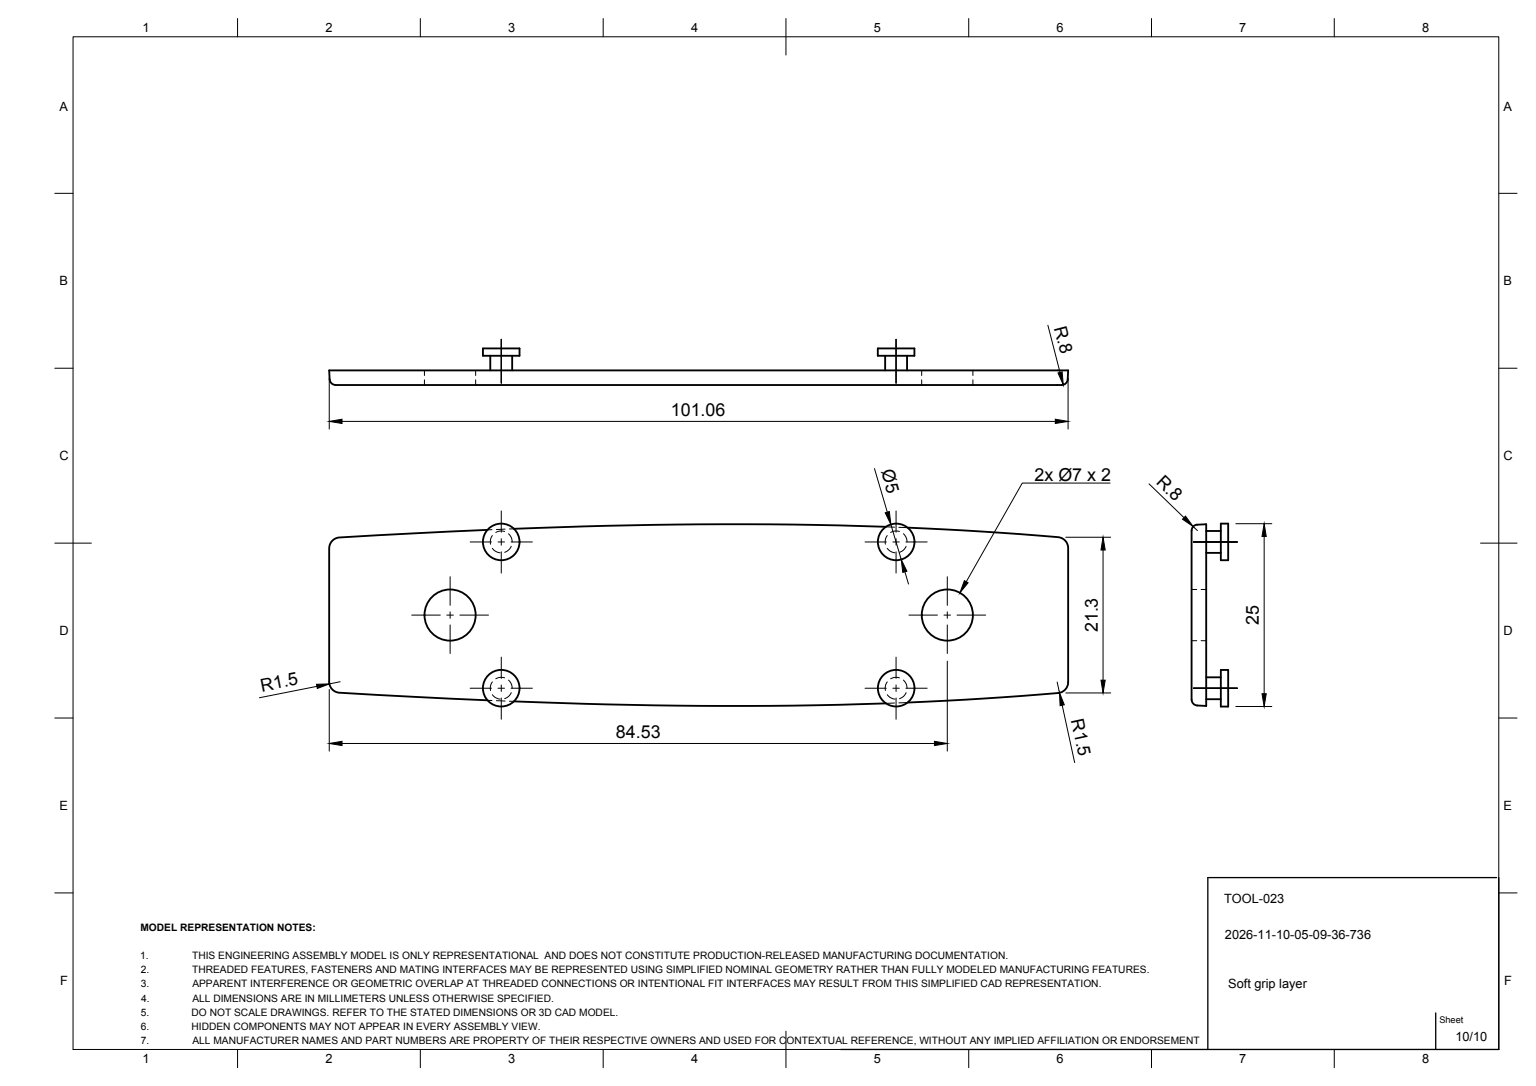
ISO-10303-21;
HEADER;
/* Generated by software containing ST-Developer
 * from STEP Tools, Inc. (www.steptools.com) 
 */

FILE_DESCRIPTION(
/* description */ (''),
/* implementation_level */ '2;1');

FILE_NAME(
/* name */ 'Soft grip layer.step',
/* time_stamp */ '2026-11-10T05:40:20-08:00',
/* author */ (''),
/* organization */ (''),
/* preprocessor_version */ 'ST-DEVELOPER v20.2',
/* originating_system */ 'Autodesk Translation Framework v15.17.0.0',
/* authorisation */ '');

FILE_SCHEMA (('AUTOMOTIVE_DESIGN { 1 0 10303 214 3 1 1 }'));
ENDSEC;

DATA;
#10=MECHANICAL_DESIGN_GEOMETRIC_PRESENTATION_REPRESENTATION('',(#579),#18580);
#160=B_SPLINE_SURFACE_WITH_KNOTS('',3,3,((#18008,#18009,#18010,#18011,#18012),
(#18013,#18014,#18015,#18016,#18017),(#18018,#18019,#18020,#18021,#18022),
(#18023,#18024,#18025,#18026,#18027),(#18028,#18029,#18030,#18031,#18032)),
 .UNSPECIFIED.,.F.,.F.,.F.,(4,1,4),(4,1,4),(0.,0.571428571428571,1.),(0.,
0.0453052401185593,0.105712226943305),.UNSPECIFIED.);
#161=B_SPLINE_SURFACE_WITH_KNOTS('',3,3,((#18055,#18056,#18057,#18058,#18059),
(#18060,#18061,#18062,#18063,#18064),(#18065,#18066,#18067,#18068,#18069),
(#18070,#18071,#18072,#18073,#18074),(#18075,#18076,#18077,#18078,#18079)),
 .UNSPECIFIED.,.F.,.F.,.F.,(4,1,4),(4,1,4),(0.,0.571428571428571,1.),(0.,
0.0453052401439183,0.105712227002476),.UNSPECIFIED.);
#162=B_SPLINE_SURFACE_WITH_KNOTS('',3,3,((#18093,#18094,#18095,#18096,#18097),
(#18098,#18099,#18100,#18101,#18102),(#18103,#18104,#18105,#18106,#18107),
(#18108,#18109,#18110,#18111,#18112),(#18113,#18114,#18115,#18116,#18117)),
 .UNSPECIFIED.,.F.,.F.,.F.,(4,1,4),(4,1,4),(0.,0.571428571428571,1.),(0.,
4.20509945658767,9.8118987320379),.UNSPECIFIED.);
#163=B_SPLINE_SURFACE_WITH_KNOTS('',3,3,((#18131,#18132,#18133,#18134,#18135),
(#18136,#18137,#18138,#18139,#18140),(#18141,#18142,#18143,#18144,#18145),
(#18146,#18147,#18148,#18149,#18150),(#18151,#18152,#18153,#18154,#18155)),
 .UNSPECIFIED.,.F.,.F.,.F.,(4,1,4),(4,1,4),(0.,0.571428571428571,1.),(0.,
0.0444882141544403,0.103805833027027),.UNSPECIFIED.);
#164=B_SPLINE_SURFACE_WITH_KNOTS('',3,3,((#18175,#18176,#18177,#18178,#18179),
(#18180,#18181,#18182,#18183,#18184),(#18185,#18186,#18187,#18188,#18189),
(#18190,#18191,#18192,#18193,#18194),(#18195,#18196,#18197,#18198,#18199)),
 .UNSPECIFIED.,.F.,.F.,.F.,(4,1,4),(4,1,4),(0.,0.571428571428571,1.),(2.06005858395869E-18,
0.0444882141931362,0.103805833117318),.UNSPECIFIED.);
#165=B_SPLINE_SURFACE_WITH_KNOTS('',3,3,((#18213,#18214,#18215,#18216,#18217),
(#18218,#18219,#18220,#18221,#18222),(#18223,#18224,#18225,#18226,#18227),
(#18228,#18229,#18230,#18231,#18232),(#18233,#18234,#18235,#18236,#18237)),
 .UNSPECIFIED.,.F.,.F.,.F.,(4,1,4),(4,1,4),(0.,0.571428571428571,1.),(0.,
4.20509909783593,9.81189789495051),.UNSPECIFIED.);
#166=B_SPLINE_SURFACE_WITH_KNOTS('',3,3,((#18260,#18261,#18262,#18263),
(#18264,#18265,#18266,#18267),(#18268,#18269,#18270,#18271),(#18272,#18273,
#18274,#18275),(#18276,#18277,#18278,#18279)),.UNSPECIFIED.,.F.,.F.,.F.,
(4,1,4),(4,4),(0.,0.571428571428571,1.),(-0.00268702576369722,0.125151053668407),
 .UNSPECIFIED.);
#167=B_SPLINE_SURFACE_WITH_KNOTS('',3,3,((#18313,#18314,#18315,#18316),
(#18317,#18318,#18319,#18320),(#18321,#18322,#18323,#18324),(#18325,#18326,
#18327,#18328)),.UNSPECIFIED.,.F.,.F.,.F.,(4,4),(4,4),(0.0135518988075539,
0.986045335056424),(0.,0.622596671418298),.UNSPECIFIED.);
#168=B_SPLINE_SURFACE_WITH_KNOTS('',3,3,((#18338,#18339,#18340,#18341),
(#18342,#18343,#18344,#18345),(#18346,#18347,#18348,#18349),(#18350,#18351,
#18352,#18353),(#18354,#18355,#18356,#18357)),.UNSPECIFIED.,.F.,.F.,.F.,
(4,1,4),(4,4),(0.,0.571428571428571,1.),(-0.00281084541253883,0.124959300034279),
 .UNSPECIFIED.);
#169=B_SPLINE_SURFACE_WITH_KNOTS('',3,3,((#18399,#18400,#18401,#18402),
(#18403,#18404,#18405,#18406),(#18407,#18408,#18409,#18410),(#18411,#18412,
#18413,#18414),(#18415,#18416,#18417,#18418)),.UNSPECIFIED.,.F.,.F.,.F.,
(4,1,4),(4,4),(0.,0.571428571428571,1.),(-0.00261432509268751,0.125151053668407),
 .UNSPECIFIED.);
#170=B_SPLINE_SURFACE_WITH_KNOTS('',3,3,((#18452,#18453,#18454,#18455),
(#18456,#18457,#18458,#18459),(#18460,#18461,#18462,#18463),(#18464,#18465,
#18466,#18467),(#18468,#18469,#18470,#18471)),.UNSPECIFIED.,.F.,.F.,.F.,
(4,1,4),(4,4),(0.,0.571428571428571,1.),(-0.00286362952972032,0.124959300034279),
 .UNSPECIFIED.);
#171=B_SPLINE_SURFACE_WITH_KNOTS('',3,3,((#18510,#18511,#18512,#18513),
(#18514,#18515,#18516,#18517),(#18518,#18519,#18520,#18521),(#18522,#18523,
#18524,#18525)),.UNSPECIFIED.,.F.,.F.,.F.,(4,4),(4,4),(0.0139546649435754,
0.986448101192446),(0.,0.622596671418299),.UNSPECIFIED.);
#528=B_SPLINE_CURVE_WITH_KNOTS('',3,(#18037,#18038,#18039,#18040,#18041),
 .UNSPECIFIED.,.F.,.F.,(4,1,4),(-0.105712226943305,-0.0453052401185593,
0.),.UNSPECIFIED.);
#529=B_SPLINE_CURVE_WITH_KNOTS('',3,(#18044,#18045,#18046,#18047,#18048),
 .UNSPECIFIED.,.F.,.F.,(4,1,4),(0.,0.0453052401185593,0.105712226943305),
 .UNSPECIFIED.);
#530=B_SPLINE_CURVE_WITH_KNOTS('',3,(#18083,#18084,#18085,#18086,#18087),
 .UNSPECIFIED.,.F.,.F.,(4,1,4),(-0.105712227002476,-0.0453052401439183,
0.),.UNSPECIFIED.);
#531=B_SPLINE_CURVE_WITH_KNOTS('',3,(#18088,#18089,#18090,#18091,#18092),
 .UNSPECIFIED.,.F.,.F.,(4,1,4),(0.,0.0453052401439183,0.105712227002476),
 .UNSPECIFIED.);
#532=B_SPLINE_CURVE_WITH_KNOTS('',3,(#18121,#18122,#18123,#18124,#18125),
 .UNSPECIFIED.,.F.,.F.,(4,1,4),(-9.8118987320379,-4.20509945658767,0.),
 .UNSPECIFIED.);
#533=B_SPLINE_CURVE_WITH_KNOTS('',3,(#18126,#18127,#18128,#18129,#18130),
 .UNSPECIFIED.,.F.,.F.,(4,1,4),(0.,4.20509945658767,9.8118987320379),
 .UNSPECIFIED.);
#534=B_SPLINE_CURVE_WITH_KNOTS('',3,(#18159,#18160,#18161,#18162,#18163),
 .UNSPECIFIED.,.F.,.F.,(4,1,4),(-0.103805833027027,-0.0444882141544403,
0.),.UNSPECIFIED.);
#535=B_SPLINE_CURVE_WITH_KNOTS('',3,(#18164,#18165,#18166,#18167,#18168),
 .UNSPECIFIED.,.F.,.F.,(4,1,4),(0.,0.0444882141544403,0.103805833027027),
 .UNSPECIFIED.);
#536=B_SPLINE_CURVE_WITH_KNOTS('',3,(#18203,#18204,#18205,#18206,#18207),
 .UNSPECIFIED.,.F.,.F.,(4,1,4),(-0.103805833117318,-0.0444882141931362,
-2.06005858395869E-18),.UNSPECIFIED.);
#537=B_SPLINE_CURVE_WITH_KNOTS('',3,(#18208,#18209,#18210,#18211,#18212),
 .UNSPECIFIED.,.F.,.F.,(4,1,4),(2.06005858395869E-18,0.0444882141931362,
0.103805833117318),.UNSPECIFIED.);
#538=B_SPLINE_CURVE_WITH_KNOTS('',3,(#18238,#18239,#18240,#18241,#18242),
 .UNSPECIFIED.,.F.,.F.,(4,1,4),(-9.81189789495051,-4.20509909783593,0.),
 .UNSPECIFIED.);
#539=B_SPLINE_CURVE_WITH_KNOTS('',3,(#18243,#18244,#18245,#18246,#18247),
 .UNSPECIFIED.,.F.,.F.,(4,1,4),(0.,4.20509909783593,9.81189789495051),
 .UNSPECIFIED.);
#540=B_SPLINE_CURVE_WITH_KNOTS('',3,(#18250,#18251,#18252,#18253),
 .UNSPECIFIED.,.F.,.F.,(4,4),(0.00062434729305816,0.125151053668407),
 .UNSPECIFIED.);
#541=B_SPLINE_CURVE_WITH_KNOTS('',3,(#18256,#18257,#18258,#18259),
 .UNSPECIFIED.,.F.,.F.,(4,4),(-0.125151053668407,-0.000624347293058304),
 .UNSPECIFIED.);
#542=B_SPLINE_CURVE_WITH_KNOTS('',3,(#18281,#18282,#18283,#18284),
 .UNSPECIFIED.,.F.,.F.,(4,4),(-0.124859357077656,3.91613824701764E-16),
 .UNSPECIFIED.);
#543=B_SPLINE_CURVE_WITH_KNOTS('',3,(#18285,#18286,#18287,#18288,#18289,
#18290,#18291,#18292,#18293,#18294,#18295,#18296,#18297,#18298,#18299,#18300,
#18301,#18302,#18303,#18304,#18305,#18306,#18307,#18308,#18309,#18310,#18311,
#18312),.UNSPECIFIED.,.F.,.F.,(4,3,3,3,3,3,3,3,3,4),(0.,0.0322709922822142,
0.0586131010579366,0.0908535483049993,0.095660418056781,0.117090121226367,
0.14947943031994,0.17008966569926,0.202270498561131,0.223122165115773),
 .UNSPECIFIED.);
#544=B_SPLINE_CURVE_WITH_KNOTS('',3,(#18330,#18331,#18332,#18333),
 .UNSPECIFIED.,.F.,.F.,(4,4),(1.57426155444895E-16,0.124757292074316),
 .UNSPECIFIED.);
#545=B_SPLINE_CURVE_WITH_KNOTS('',3,(#18334,#18335,#18336,#18337),
 .UNSPECIFIED.,.F.,.F.,(4,4),(0.0135518988075539,0.986045335056425),
 .UNSPECIFIED.);
#546=B_SPLINE_CURVE_WITH_KNOTS('',3,(#18359,#18360,#18361,#18362),
 .UNSPECIFIED.,.F.,.F.,(4,4),(-0.124959300034279,-0.000432357919845506),
 .UNSPECIFIED.);
#547=B_SPLINE_CURVE_WITH_KNOTS('',3,(#18363,#18364,#18365,#18366,#18367,
#18368,#18369,#18370,#18371,#18372,#18373,#18374,#18375,#18376,#18377,#18378,
#18379,#18380,#18381,#18382,#18383,#18384,#18385,#18386,#18387,#18388,#18389,
#18390),.UNSPECIFIED.,.F.,.F.,(4,3,3,3,3,3,3,3,3,4),(0.,0.0322720371751271,
0.0586511315716134,0.0908889384397039,0.0974306796249642,0.117149930269381,
0.149553095257184,0.172178760978465,0.204364325027201,0.227238249760569),
 .UNSPECIFIED.);
#548=B_SPLINE_CURVE_WITH_KNOTS('',3,(#18394,#18395,#18396,#18397),
 .UNSPECIFIED.,.F.,.F.,(4,4),(0.000432357919845864,0.124959300034279),
 .UNSPECIFIED.);
#549=B_SPLINE_CURVE_WITH_KNOTS('',3,(#18420,#18421,#18422,#18423,#18424,
#18425,#18426,#18427,#18428,#18429,#18430,#18431,#18432,#18433,#18434,#18435,
#18436,#18437,#18438,#18439,#18440,#18441,#18442,#18443,#18444,#18445,#18446,
#18447),.UNSPECIFIED.,.F.,.F.,(4,3,3,3,3,3,3,3,3,4),(0.,0.0322770007607458,
0.0586509099358757,0.0908890592373506,0.0956758252683957,0.117149647541228,
0.149540928065794,0.17012301918783,0.202296660223156,0.2231241621482),
 .UNSPECIFIED.);
#550=B_SPLINE_CURVE_WITH_KNOTS('',3,(#18448,#18449,#18450,#18451),
 .UNSPECIFIED.,.F.,.F.,(4,4),(1.94722710178397E-16,0.124859357077656),
 .UNSPECIFIED.);
#551=B_SPLINE_CURVE_WITH_KNOTS('',3,(#18473,#18474,#18475,#18476),
 .UNSPECIFIED.,.F.,.F.,(4,4),(-0.124757292074297,-2.43294967505747E-16),
 .UNSPECIFIED.);
#552=B_SPLINE_CURVE_WITH_KNOTS('',3,(#18477,#18478,#18479,#18480,#18481,
#18482,#18483,#18484,#18485,#18486,#18487,#18488,#18489,#18490,#18491,#18492,
#18493,#18494,#18495,#18496,#18497,#18498,#18499,#18500,#18501,#18502,#18503,
#18504),.UNSPECIFIED.,.F.,.F.,(4,3,3,3,3,3,3,3,3,4),(0.,0.0322677829554273,
0.0586251784806003,0.0908644978360146,0.097419835848357,0.117108565494702,
0.149510109206484,0.172155480916619,0.204345933772221,0.227236831322489),
 .UNSPECIFIED.);
#553=B_SPLINE_CURVE_WITH_KNOTS('',3,(#18506,#18507,#18508,#18509),
 .UNSPECIFIED.,.F.,.F.,(4,4),(0.0139546649435756,0.986448101192446),
 .UNSPECIFIED.);
#561=SHAPE_REPRESENTATION_RELATIONSHIP('SRR','None',#18632,#570);
#570=ADVANCED_BREP_SHAPE_REPRESENTATION('',(#588),#18578);
#579=STYLED_ITEM('',(#18688),#588);
#588=MANIFOLD_SOLID_BREP('Body1',#6551);
#637=FACE_BOUND('',#1558,.T.);
#638=FACE_BOUND('',#1562,.T.);
#639=FACE_BOUND('',#1566,.T.);
#640=FACE_BOUND('',#1570,.T.);
#641=FACE_BOUND('',#1590,.T.);
#642=FACE_BOUND('',#1591,.T.);
#643=FACE_BOUND('',#1596,.T.);
#644=FACE_BOUND('',#1597,.T.);
#645=FACE_BOUND('',#1598,.T.);
#646=FACE_BOUND('',#1599,.T.);
#647=FACE_BOUND('',#1600,.T.);
#648=FACE_BOUND('',#1601,.T.);
#782=PLANE('',#7063);
#783=PLANE('',#7068);
#784=PLANE('',#7069);
#785=PLANE('',#7074);
#786=PLANE('',#7075);
#787=PLANE('',#7080);
#788=PLANE('',#7081);
#789=PLANE('',#7086);
#790=PLANE('',#7105);
#791=PLANE('',#7106);
#792=PLANE('',#7107);
#793=PLANE('',#7108);
#1132=FACE_OUTER_BOUND('',#1555,.T.);
#1133=FACE_OUTER_BOUND('',#1556,.T.);
#1134=FACE_OUTER_BOUND('',#1557,.T.);
#1135=FACE_OUTER_BOUND('',#1559,.T.);
#1136=FACE_OUTER_BOUND('',#1560,.T.);
#1137=FACE_OUTER_BOUND('',#1561,.T.);
#1138=FACE_OUTER_BOUND('',#1563,.T.);
#1139=FACE_OUTER_BOUND('',#1564,.T.);
#1140=FACE_OUTER_BOUND('',#1565,.T.);
#1141=FACE_OUTER_BOUND('',#1567,.T.);
#1142=FACE_OUTER_BOUND('',#1568,.T.);
#1143=FACE_OUTER_BOUND('',#1569,.T.);
#1144=FACE_OUTER_BOUND('',#1571,.T.);
#1145=FACE_OUTER_BOUND('',#1572,.T.);
#1146=FACE_OUTER_BOUND('',#1573,.T.);
#1147=FACE_OUTER_BOUND('',#1574,.T.);
#1148=FACE_OUTER_BOUND('',#1575,.T.);
#1149=FACE_OUTER_BOUND('',#1576,.T.);
#1150=FACE_OUTER_BOUND('',#1577,.T.);
#1151=FACE_OUTER_BOUND('',#1578,.T.);
#1152=FACE_OUTER_BOUND('',#1579,.T.);
#1153=FACE_OUTER_BOUND('',#1580,.T.);
#1154=FACE_OUTER_BOUND('',#1581,.T.);
#1155=FACE_OUTER_BOUND('',#1582,.T.);
#1156=FACE_OUTER_BOUND('',#1583,.T.);
#1157=FACE_OUTER_BOUND('',#1584,.T.);
#1158=FACE_OUTER_BOUND('',#1585,.T.);
#1159=FACE_OUTER_BOUND('',#1586,.T.);
#1160=FACE_OUTER_BOUND('',#1587,.T.);
#1161=FACE_OUTER_BOUND('',#1588,.T.);
#1162=FACE_OUTER_BOUND('',#1589,.T.);
#1163=FACE_OUTER_BOUND('',#1592,.T.);
#1164=FACE_OUTER_BOUND('',#1593,.T.);
#1165=FACE_OUTER_BOUND('',#1594,.T.);
#1166=FACE_OUTER_BOUND('',#1595,.T.);
#1167=FACE_OUTER_BOUND('',#1602,.T.);
#1555=EDGE_LOOP('',(#5882,#5883,#5884,#5885));
#1556=EDGE_LOOP('',(#5886,#5887,#5888,#5889));
#1557=EDGE_LOOP('',(#5890));
#1558=EDGE_LOOP('',(#5891));
#1559=EDGE_LOOP('',(#5892,#5893,#5894,#5895));
#1560=EDGE_LOOP('',(#5896));
#1561=EDGE_LOOP('',(#5897));
#1562=EDGE_LOOP('',(#5898));
#1563=EDGE_LOOP('',(#5899,#5900,#5901,#5902));
#1564=EDGE_LOOP('',(#5903));
#1565=EDGE_LOOP('',(#5904));
#1566=EDGE_LOOP('',(#5905));
#1567=EDGE_LOOP('',(#5906,#5907,#5908,#5909));
#1568=EDGE_LOOP('',(#5910));
#1569=EDGE_LOOP('',(#5911));
#1570=EDGE_LOOP('',(#5912));
#1571=EDGE_LOOP('',(#5913,#5914,#5915,#5916));
#1572=EDGE_LOOP('',(#5917));
#1573=EDGE_LOOP('',(#5918,#5919,#5920,#5921));
#1574=EDGE_LOOP('',(#5922,#5923,#5924,#5925));
#1575=EDGE_LOOP('',(#5926,#5927,#5928,#5929));
#1576=EDGE_LOOP('',(#5930,#5931,#5932,#5933));
#1577=EDGE_LOOP('',(#5934,#5935,#5936,#5937));
#1578=EDGE_LOOP('',(#5938,#5939,#5940,#5941));
#1579=EDGE_LOOP('',(#5942,#5943,#5944,#5945));
#1580=EDGE_LOOP('',(#5946,#5947,#5948,#5949));
#1581=EDGE_LOOP('',(#5950,#5951,#5952,#5953));
#1582=EDGE_LOOP('',(#5954,#5955,#5956,#5957));
#1583=EDGE_LOOP('',(#5958,#5959,#5960,#5961));
#1584=EDGE_LOOP('',(#5962,#5963,#5964,#5965));
#1585=EDGE_LOOP('',(#5966,#5967,#5968,#5969));
#1586=EDGE_LOOP('',(#5970,#5971,#5972,#5973));
#1587=EDGE_LOOP('',(#5974,#5975,#5976,#5977));
#1588=EDGE_LOOP('',(#5978,#5979,#5980,#5981));
#1589=EDGE_LOOP('',(#5982,#5983,#5984,#5985,#5986,#5987,#5988,#5989));
#1590=EDGE_LOOP('',(#5990));
#1591=EDGE_LOOP('',(#5991));
#1592=EDGE_LOOP('',(#5992,#5993,#5994,#5995));
#1593=EDGE_LOOP('',(#5996,#5997,#5998,#5999));
#1594=EDGE_LOOP('',(#6000,#6001,#6002,#6003));
#1595=EDGE_LOOP('',(#6004,#6005,#6006,#6007,#6008,#6009,#6010,#6011));
#1596=EDGE_LOOP('',(#6012));
#1597=EDGE_LOOP('',(#6013));
#1598=EDGE_LOOP('',(#6014));
#1599=EDGE_LOOP('',(#6015));
#1600=EDGE_LOOP('',(#6016));
#1601=EDGE_LOOP('',(#6017));
#1602=EDGE_LOOP('',(#6018,#6019,#6020,#6021));
#1998=LINE('',#17944,#2405);
#1999=LINE('',#17950,#2406);
#2000=LINE('',#17960,#2407);
#2001=LINE('',#17970,#2408);
#2002=LINE('',#17980,#2409);
#2003=LINE('',#17990,#2410);
#2004=LINE('',#17994,#2411);
#2005=LINE('',#17998,#2412);
#2006=LINE('',#18002,#2413);
#2007=LINE('',#18006,#2414);
#2008=LINE('',#18053,#2415);
#2009=LINE('',#18054,#2416);
#2010=LINE('',#18173,#2417);
#2011=LINE('',#18174,#2418);
#2012=LINE('',#18255,#2419);
#2013=LINE('',#18398,#2420);
#2405=VECTOR('',#8335,0.35);
#2406=VECTOR('',#8342,0.35);
#2407=VECTOR('',#8355,0.25);
#2408=VECTOR('',#8368,0.25);
#2409=VECTOR('',#8381,0.25);
#2410=VECTOR('',#8394,0.25);
#2411=VECTOR('',#8399,0.15);
#2412=VECTOR('',#8404,0.15);
#2413=VECTOR('',#8409,0.15);
#2414=VECTOR('',#8414,0.15);
#2415=VECTOR('',#8425,1.);
#2416=VECTOR('',#8426,1.);
#2417=VECTOR('',#8437,1.);
#2418=VECTOR('',#8438,1.);
#2419=VECTOR('',#8443,1.);
#2420=VECTOR('',#8448,1.);
#2549=CIRCLE('',#7058,0.35);
#2550=CIRCLE('',#7059,0.35);
#2551=CIRCLE('',#7061,0.35);
#2552=CIRCLE('',#7062,0.35);
#2553=CIRCLE('',#7064,0.25);
#2554=CIRCLE('',#7065,0.15);
#2555=CIRCLE('',#7067,0.25);
#2556=CIRCLE('',#7070,0.25);
#2557=CIRCLE('',#7071,0.15);
#2558=CIRCLE('',#7073,0.25);
#2559=CIRCLE('',#7076,0.25);
#2560=CIRCLE('',#7077,0.15);
#2561=CIRCLE('',#7079,0.25);
#2562=CIRCLE('',#7082,0.25);
#2563=CIRCLE('',#7083,0.15);
#2564=CIRCLE('',#7085,0.25);
#2565=CIRCLE('',#7088,0.15);
#2566=CIRCLE('',#7090,0.15);
#2567=CIRCLE('',#7092,0.15);
#2568=CIRCLE('',#7094,0.15);
#2569=CIRCLE('',#7095,0.0800000000000001);
#2570=CIRCLE('',#7096,0.0799999999999999);
#2571=CIRCLE('',#7098,0.0800000000000001);
#2572=CIRCLE('',#7099,0.0800000000000001);
#2573=CIRCLE('',#7100,0.0800000000000001);
#2574=CIRCLE('',#7101,0.0800000000000001);
#2575=CIRCLE('',#7103,0.0800000000000001);
#2576=CIRCLE('',#7104,0.0800000000000001);
#3145=VERTEX_POINT('',#17941);
#3146=VERTEX_POINT('',#17943);
#3147=VERTEX_POINT('',#17947);
#3148=VERTEX_POINT('',#17949);
#3149=VERTEX_POINT('',#17953);
#3150=VERTEX_POINT('',#17955);
#3151=VERTEX_POINT('',#17958);
#3152=VERTEX_POINT('',#17963);
#3153=VERTEX_POINT('',#17965);
#3154=VERTEX_POINT('',#17968);
#3155=VERTEX_POINT('',#17973);
#3156=VERTEX_POINT('',#17975);
#3157=VERTEX_POINT('',#17978);
#3158=VERTEX_POINT('',#17983);
#3159=VERTEX_POINT('',#17985);
#3160=VERTEX_POINT('',#17988);
#3161=VERTEX_POINT('',#17993);
#3162=VERTEX_POINT('',#17997);
#3163=VERTEX_POINT('',#18001);
#3164=VERTEX_POINT('',#18005);
#3165=VERTEX_POINT('',#18033);
#3166=VERTEX_POINT('',#18034);
#3167=VERTEX_POINT('',#18036);
#3168=VERTEX_POINT('',#18042);
#3169=VERTEX_POINT('',#18050);
#3170=VERTEX_POINT('',#18051);
#3171=VERTEX_POINT('',#18080);
#3172=VERTEX_POINT('',#18081);
#3173=VERTEX_POINT('',#18118);
#3174=VERTEX_POINT('',#18119);
#3175=VERTEX_POINT('',#18156);
#3176=VERTEX_POINT('',#18157);
#3177=VERTEX_POINT('',#18170);
#3178=VERTEX_POINT('',#18171);
#3179=VERTEX_POINT('',#18200);
#3180=VERTEX_POINT('',#18201);
#3181=VERTEX_POINT('',#18249);
#3182=VERTEX_POINT('',#18254);
#3183=VERTEX_POINT('',#18280);
#3184=VERTEX_POINT('',#18329);
#3185=VERTEX_POINT('',#18358);
#3186=VERTEX_POINT('',#18393);
#3187=VERTEX_POINT('',#18419);
#3188=VERTEX_POINT('',#18472);
#4064=EDGE_CURVE('',#3145,#3145,#2549,.T.);
#4065=EDGE_CURVE('',#3145,#3146,#1998,.T.);
#4066=EDGE_CURVE('',#3146,#3146,#2550,.T.);
#4067=EDGE_CURVE('',#3147,#3147,#2551,.T.);
#4068=EDGE_CURVE('',#3147,#3148,#1999,.T.);
#4069=EDGE_CURVE('',#3148,#3148,#2552,.T.);
#4070=EDGE_CURVE('',#3149,#3149,#2553,.T.);
#4071=EDGE_CURVE('',#3150,#3150,#2554,.T.);
#4072=EDGE_CURVE('',#3151,#3151,#2555,.T.);
#4073=EDGE_CURVE('',#3151,#3149,#2000,.T.);
#4074=EDGE_CURVE('',#3152,#3152,#2556,.T.);
#4075=EDGE_CURVE('',#3153,#3153,#2557,.T.);
#4076=EDGE_CURVE('',#3154,#3154,#2558,.T.);
#4077=EDGE_CURVE('',#3154,#3152,#2001,.T.);
#4078=EDGE_CURVE('',#3155,#3155,#2559,.T.);
#4079=EDGE_CURVE('',#3156,#3156,#2560,.T.);
#4080=EDGE_CURVE('',#3157,#3157,#2561,.T.);
#4081=EDGE_CURVE('',#3157,#3155,#2002,.T.);
#4082=EDGE_CURVE('',#3158,#3158,#2562,.T.);
#4083=EDGE_CURVE('',#3159,#3159,#2563,.T.);
#4084=EDGE_CURVE('',#3160,#3160,#2564,.T.);
#4085=EDGE_CURVE('',#3160,#3158,#2003,.T.);
#4086=EDGE_CURVE('',#3150,#3161,#2004,.T.);
#4087=EDGE_CURVE('',#3161,#3161,#2565,.T.);
#4088=EDGE_CURVE('',#3153,#3162,#2005,.T.);
#4089=EDGE_CURVE('',#3162,#3162,#2566,.T.);
#4090=EDGE_CURVE('',#3156,#3163,#2006,.T.);
#4091=EDGE_CURVE('',#3163,#3163,#2567,.T.);
#4092=EDGE_CURVE('',#3159,#3164,#2007,.T.);
#4093=EDGE_CURVE('',#3164,#3164,#2568,.T.);
#4094=EDGE_CURVE('',#3165,#3166,#2569,.T.);
#4095=EDGE_CURVE('',#3166,#3167,#528,.T.);
#4096=EDGE_CURVE('',#3167,#3168,#2570,.T.);
#4097=EDGE_CURVE('',#3168,#3165,#529,.T.);
#4098=EDGE_CURVE('',#3169,#3170,#2571,.T.);
#4099=EDGE_CURVE('',#3170,#3166,#2008,.T.);
#4100=EDGE_CURVE('',#3165,#3169,#2009,.T.);
#4101=EDGE_CURVE('',#3171,#3172,#2572,.T.);
#4102=EDGE_CURVE('',#3172,#3170,#530,.T.);
#4103=EDGE_CURVE('',#3169,#3171,#531,.T.);
#4104=EDGE_CURVE('',#3173,#3174,#2573,.T.);
#4105=EDGE_CURVE('',#3174,#3172,#532,.T.);
#4106=EDGE_CURVE('',#3171,#3173,#533,.T.);
#4107=EDGE_CURVE('',#3175,#3176,#2574,.T.);
#4108=EDGE_CURVE('',#3176,#3174,#534,.T.);
#4109=EDGE_CURVE('',#3173,#3175,#535,.T.);
#4110=EDGE_CURVE('',#3177,#3178,#2575,.T.);
#4111=EDGE_CURVE('',#3178,#3176,#2010,.T.);
#4112=EDGE_CURVE('',#3175,#3177,#2011,.T.);
#4113=EDGE_CURVE('',#3179,#3180,#2576,.T.);
#4114=EDGE_CURVE('',#3180,#3178,#536,.T.);
#4115=EDGE_CURVE('',#3177,#3179,#537,.T.);
#4116=EDGE_CURVE('',#3167,#3180,#538,.T.);
#4117=EDGE_CURVE('',#3179,#3168,#539,.T.);
#4118=EDGE_CURVE('',#3181,#3178,#540,.T.);
#4119=EDGE_CURVE('',#3182,#3181,#2012,.T.);
#4120=EDGE_CURVE('',#3176,#3182,#541,.T.);
#4121=EDGE_CURVE('',#3180,#3183,#542,.T.);
#4122=EDGE_CURVE('',#3183,#3181,#543,.T.);
#4123=EDGE_CURVE('',#3184,#3167,#544,.T.);
#4124=EDGE_CURVE('',#3183,#3184,#545,.T.);
#4125=EDGE_CURVE('',#3166,#3185,#546,.T.);
#4126=EDGE_CURVE('',#3185,#3184,#547,.T.);
#4127=EDGE_CURVE('',#3186,#3170,#548,.T.);
#4128=EDGE_CURVE('',#3185,#3186,#2013,.T.);
#4129=EDGE_CURVE('',#3182,#3187,#549,.T.);
#4130=EDGE_CURVE('',#3187,#3174,#550,.T.);
#4131=EDGE_CURVE('',#3172,#3188,#551,.T.);
#4132=EDGE_CURVE('',#3188,#3186,#552,.T.);
#4133=EDGE_CURVE('',#3188,#3187,#553,.T.);
#5882=ORIENTED_EDGE('',*,*,#4064,.F.);
#5883=ORIENTED_EDGE('',*,*,#4065,.T.);
#5884=ORIENTED_EDGE('',*,*,#4066,.F.);
#5885=ORIENTED_EDGE('',*,*,#4065,.F.);
#5886=ORIENTED_EDGE('',*,*,#4067,.F.);
#5887=ORIENTED_EDGE('',*,*,#4068,.T.);
#5888=ORIENTED_EDGE('',*,*,#4069,.F.);
#5889=ORIENTED_EDGE('',*,*,#4068,.F.);
#5890=ORIENTED_EDGE('',*,*,#4070,.T.);
#5891=ORIENTED_EDGE('',*,*,#4071,.T.);
#5892=ORIENTED_EDGE('',*,*,#4072,.F.);
#5893=ORIENTED_EDGE('',*,*,#4073,.T.);
#5894=ORIENTED_EDGE('',*,*,#4070,.F.);
#5895=ORIENTED_EDGE('',*,*,#4073,.F.);
#5896=ORIENTED_EDGE('',*,*,#4072,.T.);
#5897=ORIENTED_EDGE('',*,*,#4074,.T.);
#5898=ORIENTED_EDGE('',*,*,#4075,.T.);
#5899=ORIENTED_EDGE('',*,*,#4076,.F.);
#5900=ORIENTED_EDGE('',*,*,#4077,.T.);
#5901=ORIENTED_EDGE('',*,*,#4074,.F.);
#5902=ORIENTED_EDGE('',*,*,#4077,.F.);
#5903=ORIENTED_EDGE('',*,*,#4076,.T.);
#5904=ORIENTED_EDGE('',*,*,#4078,.T.);
#5905=ORIENTED_EDGE('',*,*,#4079,.T.);
#5906=ORIENTED_EDGE('',*,*,#4080,.F.);
#5907=ORIENTED_EDGE('',*,*,#4081,.T.);
#5908=ORIENTED_EDGE('',*,*,#4078,.F.);
#5909=ORIENTED_EDGE('',*,*,#4081,.F.);
#5910=ORIENTED_EDGE('',*,*,#4080,.T.);
#5911=ORIENTED_EDGE('',*,*,#4082,.T.);
#5912=ORIENTED_EDGE('',*,*,#4083,.T.);
#5913=ORIENTED_EDGE('',*,*,#4084,.F.);
#5914=ORIENTED_EDGE('',*,*,#4085,.T.);
#5915=ORIENTED_EDGE('',*,*,#4082,.F.);
#5916=ORIENTED_EDGE('',*,*,#4085,.F.);
#5917=ORIENTED_EDGE('',*,*,#4084,.T.);
#5918=ORIENTED_EDGE('',*,*,#4071,.F.);
#5919=ORIENTED_EDGE('',*,*,#4086,.T.);
#5920=ORIENTED_EDGE('',*,*,#4087,.F.);
#5921=ORIENTED_EDGE('',*,*,#4086,.F.);
#5922=ORIENTED_EDGE('',*,*,#4075,.F.);
#5923=ORIENTED_EDGE('',*,*,#4088,.T.);
#5924=ORIENTED_EDGE('',*,*,#4089,.F.);
#5925=ORIENTED_EDGE('',*,*,#4088,.F.);
#5926=ORIENTED_EDGE('',*,*,#4079,.F.);
#5927=ORIENTED_EDGE('',*,*,#4090,.T.);
#5928=ORIENTED_EDGE('',*,*,#4091,.F.);
#5929=ORIENTED_EDGE('',*,*,#4090,.F.);
#5930=ORIENTED_EDGE('',*,*,#4083,.F.);
#5931=ORIENTED_EDGE('',*,*,#4092,.T.);
#5932=ORIENTED_EDGE('',*,*,#4093,.F.);
#5933=ORIENTED_EDGE('',*,*,#4092,.F.);
#5934=ORIENTED_EDGE('',*,*,#4094,.T.);
#5935=ORIENTED_EDGE('',*,*,#4095,.T.);
#5936=ORIENTED_EDGE('',*,*,#4096,.T.);
#5937=ORIENTED_EDGE('',*,*,#4097,.T.);
#5938=ORIENTED_EDGE('',*,*,#4098,.T.);
#5939=ORIENTED_EDGE('',*,*,#4099,.T.);
#5940=ORIENTED_EDGE('',*,*,#4094,.F.);
#5941=ORIENTED_EDGE('',*,*,#4100,.T.);
#5942=ORIENTED_EDGE('',*,*,#4101,.T.);
#5943=ORIENTED_EDGE('',*,*,#4102,.T.);
#5944=ORIENTED_EDGE('',*,*,#4098,.F.);
#5945=ORIENTED_EDGE('',*,*,#4103,.T.);
#5946=ORIENTED_EDGE('',*,*,#4104,.T.);
#5947=ORIENTED_EDGE('',*,*,#4105,.T.);
#5948=ORIENTED_EDGE('',*,*,#4101,.F.);
#5949=ORIENTED_EDGE('',*,*,#4106,.T.);
#5950=ORIENTED_EDGE('',*,*,#4107,.T.);
#5951=ORIENTED_EDGE('',*,*,#4108,.T.);
#5952=ORIENTED_EDGE('',*,*,#4104,.F.);
#5953=ORIENTED_EDGE('',*,*,#4109,.T.);
#5954=ORIENTED_EDGE('',*,*,#4110,.T.);
#5955=ORIENTED_EDGE('',*,*,#4111,.T.);
#5956=ORIENTED_EDGE('',*,*,#4107,.F.);
#5957=ORIENTED_EDGE('',*,*,#4112,.T.);
#5958=ORIENTED_EDGE('',*,*,#4113,.T.);
#5959=ORIENTED_EDGE('',*,*,#4114,.T.);
#5960=ORIENTED_EDGE('',*,*,#4110,.F.);
#5961=ORIENTED_EDGE('',*,*,#4115,.T.);
#5962=ORIENTED_EDGE('',*,*,#4096,.F.);
#5963=ORIENTED_EDGE('',*,*,#4116,.T.);
#5964=ORIENTED_EDGE('',*,*,#4113,.F.);
#5965=ORIENTED_EDGE('',*,*,#4117,.T.);
#5966=ORIENTED_EDGE('',*,*,#4111,.F.);
#5967=ORIENTED_EDGE('',*,*,#4118,.F.);
#5968=ORIENTED_EDGE('',*,*,#4119,.F.);
#5969=ORIENTED_EDGE('',*,*,#4120,.F.);
#5970=ORIENTED_EDGE('',*,*,#4114,.F.);
#5971=ORIENTED_EDGE('',*,*,#4121,.T.);
#5972=ORIENTED_EDGE('',*,*,#4122,.T.);
#5973=ORIENTED_EDGE('',*,*,#4118,.T.);
#5974=ORIENTED_EDGE('',*,*,#4116,.F.);
#5975=ORIENTED_EDGE('',*,*,#4123,.F.);
#5976=ORIENTED_EDGE('',*,*,#4124,.F.);
#5977=ORIENTED_EDGE('',*,*,#4121,.F.);
#5978=ORIENTED_EDGE('',*,*,#4095,.F.);
#5979=ORIENTED_EDGE('',*,*,#4125,.T.);
#5980=ORIENTED_EDGE('',*,*,#4126,.T.);
#5981=ORIENTED_EDGE('',*,*,#4123,.T.);
#5982=ORIENTED_EDGE('',*,*,#4097,.F.);
#5983=ORIENTED_EDGE('',*,*,#4117,.F.);
#5984=ORIENTED_EDGE('',*,*,#4115,.F.);
#5985=ORIENTED_EDGE('',*,*,#4112,.F.);
#5986=ORIENTED_EDGE('',*,*,#4109,.F.);
#5987=ORIENTED_EDGE('',*,*,#4106,.F.);
#5988=ORIENTED_EDGE('',*,*,#4103,.F.);
#5989=ORIENTED_EDGE('',*,*,#4100,.F.);
#5990=ORIENTED_EDGE('',*,*,#4064,.T.);
#5991=ORIENTED_EDGE('',*,*,#4067,.T.);
#5992=ORIENTED_EDGE('',*,*,#4099,.F.);
#5993=ORIENTED_EDGE('',*,*,#4127,.F.);
#5994=ORIENTED_EDGE('',*,*,#4128,.F.);
#5995=ORIENTED_EDGE('',*,*,#4125,.F.);
#5996=ORIENTED_EDGE('',*,*,#4108,.F.);
#5997=ORIENTED_EDGE('',*,*,#4120,.T.);
#5998=ORIENTED_EDGE('',*,*,#4129,.T.);
#5999=ORIENTED_EDGE('',*,*,#4130,.T.);
#6000=ORIENTED_EDGE('',*,*,#4102,.F.);
#6001=ORIENTED_EDGE('',*,*,#4131,.T.);
#6002=ORIENTED_EDGE('',*,*,#4132,.T.);
#6003=ORIENTED_EDGE('',*,*,#4127,.T.);
#6004=ORIENTED_EDGE('',*,*,#4126,.F.);
#6005=ORIENTED_EDGE('',*,*,#4128,.T.);
#6006=ORIENTED_EDGE('',*,*,#4132,.F.);
#6007=ORIENTED_EDGE('',*,*,#4133,.T.);
#6008=ORIENTED_EDGE('',*,*,#4129,.F.);
#6009=ORIENTED_EDGE('',*,*,#4119,.T.);
#6010=ORIENTED_EDGE('',*,*,#4122,.F.);
#6011=ORIENTED_EDGE('',*,*,#4124,.T.);
#6012=ORIENTED_EDGE('',*,*,#4066,.T.);
#6013=ORIENTED_EDGE('',*,*,#4069,.T.);
#6014=ORIENTED_EDGE('',*,*,#4087,.T.);
#6015=ORIENTED_EDGE('',*,*,#4089,.T.);
#6016=ORIENTED_EDGE('',*,*,#4091,.T.);
#6017=ORIENTED_EDGE('',*,*,#4093,.T.);
#6018=ORIENTED_EDGE('',*,*,#4105,.F.);
#6019=ORIENTED_EDGE('',*,*,#4130,.F.);
#6020=ORIENTED_EDGE('',*,*,#4133,.F.);
#6021=ORIENTED_EDGE('',*,*,#4131,.F.);
#6154=CYLINDRICAL_SURFACE('',#7057,0.35);
#6155=CYLINDRICAL_SURFACE('',#7060,0.35);
#6156=CYLINDRICAL_SURFACE('',#7066,0.25);
#6157=CYLINDRICAL_SURFACE('',#7072,0.25);
#6158=CYLINDRICAL_SURFACE('',#7078,0.25);
#6159=CYLINDRICAL_SURFACE('',#7084,0.25);
#6160=CYLINDRICAL_SURFACE('',#7087,0.15);
#6161=CYLINDRICAL_SURFACE('',#7089,0.15);
#6162=CYLINDRICAL_SURFACE('',#7091,0.15);
#6163=CYLINDRICAL_SURFACE('',#7093,0.15);
#6164=CYLINDRICAL_SURFACE('',#7097,0.08);
#6165=CYLINDRICAL_SURFACE('',#7102,0.08);
#6504=ADVANCED_FACE('',(#1132),#6154,.F.);
#6505=ADVANCED_FACE('',(#1133),#6155,.F.);
#6506=ADVANCED_FACE('',(#1134,#637),#782,.T.);
#6507=ADVANCED_FACE('',(#1135),#6156,.T.);
#6508=ADVANCED_FACE('',(#1136),#783,.F.);
#6509=ADVANCED_FACE('',(#1137,#638),#784,.T.);
#6510=ADVANCED_FACE('',(#1138),#6157,.T.);
#6511=ADVANCED_FACE('',(#1139),#785,.F.);
#6512=ADVANCED_FACE('',(#1140,#639),#786,.T.);
#6513=ADVANCED_FACE('',(#1141),#6158,.T.);
#6514=ADVANCED_FACE('',(#1142),#787,.F.);
#6515=ADVANCED_FACE('',(#1143,#640),#788,.T.);
#6516=ADVANCED_FACE('',(#1144),#6159,.T.);
#6517=ADVANCED_FACE('',(#1145),#789,.F.);
#6518=ADVANCED_FACE('',(#1146),#6160,.T.);
#6519=ADVANCED_FACE('',(#1147),#6161,.T.);
#6520=ADVANCED_FACE('',(#1148),#6162,.T.);
#6521=ADVANCED_FACE('',(#1149),#6163,.T.);
#6522=ADVANCED_FACE('',(#1150),#160,.F.);
#6523=ADVANCED_FACE('',(#1151),#6164,.T.);
#6524=ADVANCED_FACE('',(#1152),#161,.F.);
#6525=ADVANCED_FACE('',(#1153),#162,.F.);
#6526=ADVANCED_FACE('',(#1154),#163,.F.);
#6527=ADVANCED_FACE('',(#1155),#6165,.T.);
#6528=ADVANCED_FACE('',(#1156),#164,.F.);
#6529=ADVANCED_FACE('',(#1157),#165,.F.);
#6530=ADVANCED_FACE('',(#1158),#790,.F.);
#6531=ADVANCED_FACE('',(#1159),#166,.F.);
#6532=ADVANCED_FACE('',(#1160),#167,.F.);
#6533=ADVANCED_FACE('',(#1161),#168,.F.);
#6534=ADVANCED_FACE('',(#1162,#641,#642),#791,.T.);
#6535=ADVANCED_FACE('',(#1163),#792,.F.);
#6536=ADVANCED_FACE('',(#1164),#169,.F.);
#6537=ADVANCED_FACE('',(#1165),#170,.F.);
#6538=ADVANCED_FACE('',(#1166,#643,#644,#645,#646,#647,#648),#793,.F.);
#6539=ADVANCED_FACE('',(#1167),#171,.F.);
#6551=CLOSED_SHELL('',(#6504,#6505,#6506,#6507,#6508,#6509,#6510,#6511,
#6512,#6513,#6514,#6515,#6516,#6517,#6518,#6519,#6520,#6521,#6522,#6523,
#6524,#6525,#6526,#6527,#6528,#6529,#6530,#6531,#6532,#6533,#6534,#6535,
#6536,#6537,#6538,#6539));
#7056=AXIS2_PLACEMENT_3D('',#17939,#8329,#8330);
#7057=AXIS2_PLACEMENT_3D('',#17940,#8331,#8332);
#7058=AXIS2_PLACEMENT_3D('',#17942,#8333,#8334);
#7059=AXIS2_PLACEMENT_3D('',#17945,#8336,#8337);
#7060=AXIS2_PLACEMENT_3D('',#17946,#8338,#8339);
#7061=AXIS2_PLACEMENT_3D('',#17948,#8340,#8341);
#7062=AXIS2_PLACEMENT_3D('',#17951,#8343,#8344);
#7063=AXIS2_PLACEMENT_3D('',#17952,#8345,#8346);
#7064=AXIS2_PLACEMENT_3D('',#17954,#8347,#8348);
#7065=AXIS2_PLACEMENT_3D('',#17956,#8349,#8350);
#7066=AXIS2_PLACEMENT_3D('',#17957,#8351,#8352);
#7067=AXIS2_PLACEMENT_3D('',#17959,#8353,#8354);
#7068=AXIS2_PLACEMENT_3D('',#17961,#8356,#8357);
#7069=AXIS2_PLACEMENT_3D('',#17962,#8358,#8359);
#7070=AXIS2_PLACEMENT_3D('',#17964,#8360,#8361);
#7071=AXIS2_PLACEMENT_3D('',#17966,#8362,#8363);
#7072=AXIS2_PLACEMENT_3D('',#17967,#8364,#8365);
#7073=AXIS2_PLACEMENT_3D('',#17969,#8366,#8367);
#7074=AXIS2_PLACEMENT_3D('',#17971,#8369,#8370);
#7075=AXIS2_PLACEMENT_3D('',#17972,#8371,#8372);
#7076=AXIS2_PLACEMENT_3D('',#17974,#8373,#8374);
#7077=AXIS2_PLACEMENT_3D('',#17976,#8375,#8376);
#7078=AXIS2_PLACEMENT_3D('',#17977,#8377,#8378);
#7079=AXIS2_PLACEMENT_3D('',#17979,#8379,#8380);
#7080=AXIS2_PLACEMENT_3D('',#17981,#8382,#8383);
#7081=AXIS2_PLACEMENT_3D('',#17982,#8384,#8385);
#7082=AXIS2_PLACEMENT_3D('',#17984,#8386,#8387);
#7083=AXIS2_PLACEMENT_3D('',#17986,#8388,#8389);
#7084=AXIS2_PLACEMENT_3D('',#17987,#8390,#8391);
#7085=AXIS2_PLACEMENT_3D('',#17989,#8392,#8393);
#7086=AXIS2_PLACEMENT_3D('',#17991,#8395,#8396);
#7087=AXIS2_PLACEMENT_3D('',#17992,#8397,#8398);
#7088=AXIS2_PLACEMENT_3D('',#17995,#8400,#8401);
#7089=AXIS2_PLACEMENT_3D('',#17996,#8402,#8403);
#7090=AXIS2_PLACEMENT_3D('',#17999,#8405,#8406);
#7091=AXIS2_PLACEMENT_3D('',#18000,#8407,#8408);
#7092=AXIS2_PLACEMENT_3D('',#18003,#8410,#8411);
#7093=AXIS2_PLACEMENT_3D('',#18004,#8412,#8413);
#7094=AXIS2_PLACEMENT_3D('',#18007,#8415,#8416);
#7095=AXIS2_PLACEMENT_3D('',#18035,#8417,#8418);
#7096=AXIS2_PLACEMENT_3D('',#18043,#8419,#8420);
#7097=AXIS2_PLACEMENT_3D('',#18049,#8421,#8422);
#7098=AXIS2_PLACEMENT_3D('',#18052,#8423,#8424);
#7099=AXIS2_PLACEMENT_3D('',#18082,#8427,#8428);
#7100=AXIS2_PLACEMENT_3D('',#18120,#8429,#8430);
#7101=AXIS2_PLACEMENT_3D('',#18158,#8431,#8432);
#7102=AXIS2_PLACEMENT_3D('',#18169,#8433,#8434);
#7103=AXIS2_PLACEMENT_3D('',#18172,#8435,#8436);
#7104=AXIS2_PLACEMENT_3D('',#18202,#8439,#8440);
#7105=AXIS2_PLACEMENT_3D('',#18248,#8441,#8442);
#7106=AXIS2_PLACEMENT_3D('',#18391,#8444,#8445);
#7107=AXIS2_PLACEMENT_3D('',#18392,#8446,#8447);
#7108=AXIS2_PLACEMENT_3D('',#18505,#8449,#8450);
#8329=DIRECTION('axis',(0.,0.,1.));
#8330=DIRECTION('refdir',(1.,0.,0.));
#8331=DIRECTION('center_axis',(0.,0.,-1.));
#8332=DIRECTION('ref_axis',(1.,0.,0.));
#8333=DIRECTION('center_axis',(1.16928610669829E-31,-5.97538301968883E-32,
-1.));
#8334=DIRECTION('ref_axis',(1.,0.,0.));
#8335=DIRECTION('',(0.,0.,-1.));
#8336=DIRECTION('center_axis',(-6.45616000593692E-32,-1.81182428107391E-19,
1.));
#8337=DIRECTION('ref_axis',(1.,0.,0.));
#8338=DIRECTION('center_axis',(0.,0.,-1.));
#8339=DIRECTION('ref_axis',(1.,0.,0.));
#8340=DIRECTION('center_axis',(1.16928610669829E-31,-5.97538301968883E-32,
-1.));
#8341=DIRECTION('ref_axis',(1.,0.,0.));
#8342=DIRECTION('',(0.,0.,-1.));
#8343=DIRECTION('center_axis',(-6.45616000593692E-32,-1.81182428107391E-19,
1.));
#8344=DIRECTION('ref_axis',(1.,0.,0.));
#8345=DIRECTION('center_axis',(0.,0.,1.));
#8346=DIRECTION('ref_axis',(1.,0.,0.));
#8347=DIRECTION('center_axis',(0.,0.,1.));
#8348=DIRECTION('ref_axis',(1.,0.,0.));
#8349=DIRECTION('center_axis',(0.,0.,-1.));
#8350=DIRECTION('ref_axis',(1.,0.,0.));
#8351=DIRECTION('center_axis',(0.,0.,-1.));
#8352=DIRECTION('ref_axis',(1.,0.,0.));
#8353=DIRECTION('center_axis',(0.,0.,-1.));
#8354=DIRECTION('ref_axis',(1.,0.,0.));
#8355=DIRECTION('',(0.,0.,1.));
#8356=DIRECTION('center_axis',(0.,0.,1.));
#8357=DIRECTION('ref_axis',(1.,0.,0.));
#8358=DIRECTION('center_axis',(0.,0.,1.));
#8359=DIRECTION('ref_axis',(1.,0.,0.));
#8360=DIRECTION('center_axis',(0.,0.,1.));
#8361=DIRECTION('ref_axis',(1.,0.,0.));
#8362=DIRECTION('center_axis',(0.,0.,-1.));
#8363=DIRECTION('ref_axis',(1.,0.,0.));
#8364=DIRECTION('center_axis',(0.,0.,-1.));
#8365=DIRECTION('ref_axis',(1.,0.,0.));
#8366=DIRECTION('center_axis',(0.,0.,-1.));
#8367=DIRECTION('ref_axis',(1.,0.,0.));
#8368=DIRECTION('',(0.,0.,1.));
#8369=DIRECTION('center_axis',(0.,0.,1.));
#8370=DIRECTION('ref_axis',(1.,0.,0.));
#8371=DIRECTION('center_axis',(0.,0.,1.));
#8372=DIRECTION('ref_axis',(1.,0.,0.));
#8373=DIRECTION('center_axis',(0.,0.,1.));
#8374=DIRECTION('ref_axis',(1.,0.,0.));
#8375=DIRECTION('center_axis',(0.,0.,-1.));
#8376=DIRECTION('ref_axis',(1.,0.,0.));
#8377=DIRECTION('center_axis',(0.,0.,-1.));
#8378=DIRECTION('ref_axis',(1.,0.,0.));
#8379=DIRECTION('center_axis',(0.,0.,-1.));
#8380=DIRECTION('ref_axis',(1.,0.,0.));
#8381=DIRECTION('',(0.,0.,1.));
#8382=DIRECTION('center_axis',(0.,0.,1.));
#8383=DIRECTION('ref_axis',(1.,0.,0.));
#8384=DIRECTION('center_axis',(0.,0.,1.));
#8385=DIRECTION('ref_axis',(1.,0.,0.));
#8386=DIRECTION('center_axis',(0.,0.,1.));
#8387=DIRECTION('ref_axis',(1.,0.,0.));
#8388=DIRECTION('center_axis',(0.,0.,-1.));
#8389=DIRECTION('ref_axis',(1.,0.,0.));
#8390=DIRECTION('center_axis',(0.,0.,-1.));
#8391=DIRECTION('ref_axis',(1.,0.,0.));
#8392=DIRECTION('center_axis',(0.,0.,-1.));
#8393=DIRECTION('ref_axis',(1.,0.,0.));
#8394=DIRECTION('',(0.,0.,1.));
#8395=DIRECTION('center_axis',(0.,0.,1.));
#8396=DIRECTION('ref_axis',(1.,0.,0.));
#8397=DIRECTION('center_axis',(0.,0.,-1.));
#8398=DIRECTION('ref_axis',(1.,0.,0.));
#8399=DIRECTION('',(0.,0.,1.));
#8400=DIRECTION('center_axis',(-6.45616000593692E-32,-1.81182428107391E-19,
1.));
#8401=DIRECTION('ref_axis',(1.,0.,0.));
#8402=DIRECTION('center_axis',(0.,0.,-1.));
#8403=DIRECTION('ref_axis',(1.,0.,0.));
#8404=DIRECTION('',(0.,0.,1.));
#8405=DIRECTION('center_axis',(-6.45616000593692E-32,-1.81182428107391E-19,
1.));
#8406=DIRECTION('ref_axis',(1.,0.,0.));
#8407=DIRECTION('center_axis',(0.,0.,-1.));
#8408=DIRECTION('ref_axis',(1.,0.,0.));
#8409=DIRECTION('',(0.,0.,1.));
#8410=DIRECTION('center_axis',(-6.45616000593692E-32,-1.81182428107391E-19,
1.));
#8411=DIRECTION('ref_axis',(1.,0.,0.));
#8412=DIRECTION('center_axis',(0.,0.,-1.));
#8413=DIRECTION('ref_axis',(1.,0.,0.));
#8414=DIRECTION('',(0.,0.,1.));
#8415=DIRECTION('center_axis',(-6.45616000593692E-32,-1.81182428107391E-19,
1.));
#8416=DIRECTION('ref_axis',(1.,0.,0.));
#8417=DIRECTION('center_axis',(0.,1.,0.));
#8418=DIRECTION('ref_axis',(0.,0.,1.));
#8419=DIRECTION('center_axis',(0.998287351281347,-0.0585009766728139,0.));
#8420=DIRECTION('ref_axis',(0.0584117362954384,0.996764512774636,0.0552139034672828));
#8421=DIRECTION('center_axis',(-3.13156554427463E-33,-1.,5.97538301968883E-32));
#8422=DIRECTION('ref_axis',(0.688354575693766,0.,0.725374371012276));
#8423=DIRECTION('center_axis',(1.38968329343724E-15,1.,0.));
#8424=DIRECTION('ref_axis',(0.,0.,1.));
#8425=DIRECTION('',(3.13156554427463E-33,1.,-5.97538301968883E-32));
#8426=DIRECTION('',(-3.13156554427463E-33,-1.,5.97538301968883E-32));
#8427=DIRECTION('center_axis',(0.998287351281345,0.0585009766728351,0.));
#8428=DIRECTION('ref_axis',(0.,0.,1.));
#8429=DIRECTION('center_axis',(0.996325437245183,-0.0856482521607663,0.));
#8430=DIRECTION('ref_axis',(0.,0.,1.));
#8431=DIRECTION('center_axis',(-1.38968329343725E-15,-1.,-6.75000545323542E-30));
#8432=DIRECTION('ref_axis',(-4.85722573273506E-15,0.,1.));
#8433=DIRECTION('center_axis',(-3.13156554427485E-33,1.,-5.97538301968883E-32));
#8434=DIRECTION('ref_axis',(-0.688354575693752,0.,0.72537437101229));
#8435=DIRECTION('center_axis',(1.38968329343726E-15,-1.,0.));
#8436=DIRECTION('ref_axis',(0.,0.,1.));
#8437=DIRECTION('',(3.13156554427485E-33,-1.,5.97538301968883E-32));
#8438=DIRECTION('',(-3.13156554427485E-33,1.,-5.97538301968883E-32));
#8439=DIRECTION('center_axis',(-0.996325437245184,-0.0856482521607654,-4.83937755196581E-15));
#8440=DIRECTION('ref_axis',(-4.85722573273506E-15,0.,1.));
#8441=DIRECTION('center_axis',(0.998629534754574,0.,-0.0523359562429439));
#8442=DIRECTION('ref_axis',(-0.0523359562429439,0.,-0.998629534754574));
#8443=DIRECTION('',(0.,1.,0.));
#8444=DIRECTION('center_axis',(-1.16928610669829E-31,5.97538301968883E-32,
1.));
#8445=DIRECTION('ref_axis',(1.,0.,1.16928610669829E-31));
#8446=DIRECTION('center_axis',(-0.998629534754574,0.,-0.0523359562429402));
#8447=DIRECTION('ref_axis',(-0.0523359562429402,0.,0.998629534754574));
#8448=DIRECTION('',(0.,-1.,0.));
#8449=DIRECTION('center_axis',(-6.45616000593692E-32,-1.81182428107391E-19,
1.));
#8450=DIRECTION('ref_axis',(1.,0.,6.45616000593692E-32));
#17939=CARTESIAN_POINT('',(0.,0.,0.));
#17940=CARTESIAN_POINT('Origin',(2.,0.,1.));
#17941=CARTESIAN_POINT('',(1.65,4.28626379701574E-17,1.1));
#17942=CARTESIAN_POINT('Origin',(2.,0.,1.1));
#17943=CARTESIAN_POINT('',(1.65,4.28626379701574E-17,0.9));
#17944=CARTESIAN_POINT('',(1.65,4.28626379701574E-17,1.));
#17945=CARTESIAN_POINT('Origin',(2.,0.,0.9));
#17946=CARTESIAN_POINT('Origin',(8.8,0.,1.));
#17947=CARTESIAN_POINT('',(8.45,4.28626379701574E-17,1.1));
#17948=CARTESIAN_POINT('Origin',(8.8,0.,1.1));
#17949=CARTESIAN_POINT('',(8.45,4.28626379701574E-17,0.9));
#17950=CARTESIAN_POINT('',(8.45,4.28626379701574E-17,1.));
#17951=CARTESIAN_POINT('Origin',(8.8,0.,0.9));
#17952=CARTESIAN_POINT('Origin',(8.1,1.,0.7));
#17953=CARTESIAN_POINT('',(7.85,1.,0.7));
#17954=CARTESIAN_POINT('Origin',(8.1,1.,0.7));
#17955=CARTESIAN_POINT('',(7.95,1.,0.7));
#17956=CARTESIAN_POINT('Origin',(8.1,1.,0.7));
#17957=CARTESIAN_POINT('Origin',(8.1,1.,0.7));
#17958=CARTESIAN_POINT('',(7.85,1.,0.6));
#17959=CARTESIAN_POINT('Origin',(8.1,1.,0.6));
#17960=CARTESIAN_POINT('',(7.85,1.,0.7));
#17961=CARTESIAN_POINT('Origin',(8.1,1.,0.6));
#17962=CARTESIAN_POINT('Origin',(2.7,-1.,0.7));
#17963=CARTESIAN_POINT('',(2.45,-1.,0.7));
#17964=CARTESIAN_POINT('Origin',(2.7,-1.,0.7));
#17965=CARTESIAN_POINT('',(2.55,-1.,0.7));
#17966=CARTESIAN_POINT('Origin',(2.7,-1.,0.7));
#17967=CARTESIAN_POINT('Origin',(2.7,-1.,0.7));
#17968=CARTESIAN_POINT('',(2.45,-1.,0.6));
#17969=CARTESIAN_POINT('Origin',(2.7,-1.,0.6));
#17970=CARTESIAN_POINT('',(2.45,-1.,0.7));
#17971=CARTESIAN_POINT('Origin',(2.7,-1.,0.6));
#17972=CARTESIAN_POINT('Origin',(2.7,1.,0.7));
#17973=CARTESIAN_POINT('',(2.45,1.,0.7));
#17974=CARTESIAN_POINT('Origin',(2.7,1.,0.7));
#17975=CARTESIAN_POINT('',(2.55,1.,0.7));
#17976=CARTESIAN_POINT('Origin',(2.7,1.,0.7));
#17977=CARTESIAN_POINT('Origin',(2.7,1.,0.7));
#17978=CARTESIAN_POINT('',(2.45,1.,0.6));
#17979=CARTESIAN_POINT('Origin',(2.7,1.,0.6));
#17980=CARTESIAN_POINT('',(2.45,1.,0.7));
#17981=CARTESIAN_POINT('Origin',(2.7,1.,0.6));
#17982=CARTESIAN_POINT('Origin',(8.1,-1.,0.7));
#17983=CARTESIAN_POINT('',(7.85,-1.,0.7));
#17984=CARTESIAN_POINT('Origin',(8.1,-1.,0.7));
#17985=CARTESIAN_POINT('',(7.95,-1.,0.7));
#17986=CARTESIAN_POINT('Origin',(8.1,-1.,0.7));
#17987=CARTESIAN_POINT('Origin',(8.1,-1.,0.7));
#17988=CARTESIAN_POINT('',(7.85,-1.,0.6));
#17989=CARTESIAN_POINT('Origin',(8.1,-1.,0.6));
#17990=CARTESIAN_POINT('',(7.85,-1.,0.7));
#17991=CARTESIAN_POINT('Origin',(8.1,-1.,0.6));
#17992=CARTESIAN_POINT('Origin',(8.1,1.,0.9));
#17993=CARTESIAN_POINT('',(7.95,1.,0.9));
#17994=CARTESIAN_POINT('',(7.95,1.,0.9));
#17995=CARTESIAN_POINT('Origin',(8.1,1.,0.9));
#17996=CARTESIAN_POINT('Origin',(2.7,-1.,0.9));
#17997=CARTESIAN_POINT('',(2.55,-1.,0.9));
#17998=CARTESIAN_POINT('',(2.55,-1.,0.9));
#17999=CARTESIAN_POINT('Origin',(2.7,-1.,0.9));
#18000=CARTESIAN_POINT('Origin',(2.7,1.,0.9));
#18001=CARTESIAN_POINT('',(2.55,1.,0.9));
#18002=CARTESIAN_POINT('',(2.55,1.,0.9));
#18003=CARTESIAN_POINT('Origin',(2.7,1.,0.9));
#18004=CARTESIAN_POINT('Origin',(8.1,-1.,0.9));
#18005=CARTESIAN_POINT('',(7.95,-1.,0.9));
#18006=CARTESIAN_POINT('',(7.95,-1.,0.9));
#18007=CARTESIAN_POINT('Origin',(8.1,-1.,0.9));
#18008=CARTESIAN_POINT('Ctrl Pts',(10.3006295894369,0.974894988741159,1.1));
#18009=CARTESIAN_POINT('Ctrl Pts',(10.315705472156,0.974011521809381,1.1));
#18010=CARTESIAN_POINT('Ctrl Pts',(10.3502474882039,0.960160784532573,1.1));
#18011=CARTESIAN_POINT('Ctrl Pts',(10.3664342774515,0.92524659453289,1.1));
#18012=CARTESIAN_POINT('Ctrl Pts',(10.3664342774515,0.905110932257975,1.1));
#18013=CARTESIAN_POINT('Ctrl Pts',(10.3019806204244,0.997949597787003,1.1));
#18014=CARTESIAN_POINT('Ctrl Pts',(10.3220349090938,0.996609784625678,1.09999398337427));
#18015=CARTESIAN_POINT('Ctrl Pts',(10.3677183242066,0.978025516808524,1.09998506712737));
#18016=CARTESIAN_POINT('Ctrl Pts',(10.3893396302527,0.931918448901421,1.09999143472557));
#18017=CARTESIAN_POINT('Ctrl Pts',(10.3895723566779,0.905110932257975,1.1));
#18018=CARTESIAN_POINT('Ctrl Pts',(10.3043223099121,1.03790925537118,1.08136572286424));
#18019=CARTESIAN_POINT('Ctrl Pts',(10.3329503749445,1.0358015962555,1.08164234815929));
#18020=CARTESIAN_POINT('Ctrl Pts',(10.3979372989902,1.00899285190124,1.08203919297574));
#18021=CARTESIAN_POINT('Ctrl Pts',(10.4290660105163,0.943405843911333,1.08168333012239));
#18022=CARTESIAN_POINT('Ctrl Pts',(10.4296737498558,0.905110932257975,1.08129070628762));
#18023=CARTESIAN_POINT('Ctrl Pts',(10.3052465815697,1.05368144854439,1.04171131144128));
#18024=CARTESIAN_POINT('Ctrl Pts',(10.3373036016374,1.05157771141627,1.04242733672965));
#18025=CARTESIAN_POINT('Ctrl Pts',(10.4104769365187,1.02185126978705,1.04346621563788));
#18026=CARTESIAN_POINT('Ctrl Pts',(10.445100550936,0.94795146444073,1.04253150017828));
#18027=CARTESIAN_POINT('Ctrl Pts',(10.4454164251054,0.905110932257975,1.0415166534692));
#18028=CARTESIAN_POINT('Ctrl Pts',(10.3053025283406,1.05463614976313,1.02441711227736));
#18029=CARTESIAN_POINT('Ctrl Pts',(10.3375636805833,1.05269876817044,1.02526261130878));
#18030=CARTESIAN_POINT('Ctrl Pts',(10.411517621087,1.0229540574362,1.02649649899074));
#18031=CARTESIAN_POINT('Ctrl Pts',(10.4462618831994,0.948196125723061,1.02538435201347));
#18032=CARTESIAN_POINT('Ctrl Pts',(10.4463246402318,0.905110932257975,1.02418687649944));
#18033=CARTESIAN_POINT('',(10.3664342774515,0.905110932257975,1.1));
#18034=CARTESIAN_POINT('',(10.4463246402318,0.905110932257975,1.02418687649943));
#18035=CARTESIAN_POINT('Origin',(10.3664342774515,0.905110932257975,1.02));
#18036=CARTESIAN_POINT('',(10.3053025283406,1.05463614976313,1.02441711227738));
#18037=CARTESIAN_POINT('Ctrl Pts',(10.4463246402318,0.905110932257975,1.02418687649944));
#18038=CARTESIAN_POINT('Ctrl Pts',(10.4462618831994,0.948196125723061,1.02538435201347));
#18039=CARTESIAN_POINT('Ctrl Pts',(10.411517621087,1.0229540574362,1.02649649899074));
#18040=CARTESIAN_POINT('Ctrl Pts',(10.3375636805833,1.05269876817044,1.02526261130878));
#18041=CARTESIAN_POINT('Ctrl Pts',(10.3053025283406,1.05463614976313,1.02441711227736));
#18042=CARTESIAN_POINT('',(10.3006295894369,0.974894988741159,1.1));
#18043=CARTESIAN_POINT('Origin',(10.3006295894369,0.974894988741159,1.02));
#18044=CARTESIAN_POINT('Ctrl Pts',(10.3006295894369,0.974894988741159,1.1));
#18045=CARTESIAN_POINT('Ctrl Pts',(10.315705472156,0.974011521809381,1.1));
#18046=CARTESIAN_POINT('Ctrl Pts',(10.3502474882039,0.960160784532573,1.1));
#18047=CARTESIAN_POINT('Ctrl Pts',(10.3664342774515,0.92524659453289,1.1));
#18048=CARTESIAN_POINT('Ctrl Pts',(10.3664342774515,0.905110932257975,1.1));
#18049=CARTESIAN_POINT('Origin',(10.3664342774515,0.526416499322631,1.02));
#18050=CARTESIAN_POINT('',(10.3664342774515,-0.905110932257974,1.1));
#18051=CARTESIAN_POINT('',(10.4463246402318,-0.905110932257974,1.02418687649944));
#18052=CARTESIAN_POINT('Origin',(10.3664342774515,-0.905110932257974,1.02));
#18053=CARTESIAN_POINT('',(10.4463246402318,0.526416499322631,1.02418687649944));
#18054=CARTESIAN_POINT('',(10.3664342774515,0.526416499322631,1.1));
#18055=CARTESIAN_POINT('Ctrl Pts',(10.3664342774515,-0.905110932257974,
1.1));
#18056=CARTESIAN_POINT('Ctrl Pts',(10.3664342774515,-0.920212678972614,
1.1));
#18057=CARTESIAN_POINT('Ctrl Pts',(10.3546350195413,-0.955507038097987,
1.1));
#18058=CARTESIAN_POINT('Ctrl Pts',(10.3207307664069,-0.973717032831462,
1.1));
#18059=CARTESIAN_POINT('Ctrl Pts',(10.3006295894369,-0.974894988741159,
1.1));
#18060=CARTESIAN_POINT('Ctrl Pts',(10.3895723566779,-0.905110932257974,
1.1));
#18061=CARTESIAN_POINT('Ctrl Pts',(10.3893978118589,-0.925216569751813,
1.09999357604418));
#18062=CARTESIAN_POINT('Ctrl Pts',(10.3734893817427,-0.971910228734234,
1.09998467394719));
#18063=CARTESIAN_POINT('Ctrl Pts',(10.3287196719985,-0.996163180237569,
1.09999197783236));
#18064=CARTESIAN_POINT('Ctrl Pts',(10.3019806204244,-0.997949597787003,
1.1));
#18065=CARTESIAN_POINT('Ctrl Pts',(10.4296737498558,-0.905110932257974,
1.0812907062876));
#18066=CARTESIAN_POINT('Ctrl Pts',(10.4292179453509,-0.933832116014069,
1.08158517416384));
#18067=CARTESIAN_POINT('Ctrl Pts',(10.4061705706524,-1.00027633256302,1.08203447943735));
#18068=CARTESIAN_POINT('Ctrl Pts',(10.3424930633099,-1.03509904321534,1.08173455659116));
#18069=CARTESIAN_POINT('Ctrl Pts',(10.3043223099121,-1.03790925537115,1.08136572286421));
#18070=CARTESIAN_POINT('Ctrl Pts',(10.4454164251054,-0.905110932257974,
1.0415166534692));
#18071=CARTESIAN_POINT('Ctrl Pts',(10.4451795194782,-0.937241331413026,
1.04227778850144));
#18072=CARTESIAN_POINT('Ctrl Pts',(10.4197512278104,-1.01202259423409,1.0434534732467));
#18073=CARTESIAN_POINT('Ctrl Pts',(10.3479892750172,-1.05087646570533,1.0426660118263));
#18074=CARTESIAN_POINT('Ctrl Pts',(10.3052465815697,-1.05368144854438,1.04171131144128));
#18075=CARTESIAN_POINT('Ctrl Pts',(10.4463246402318,-0.905110932257974,
1.02418687649944));
#18076=CARTESIAN_POINT('Ctrl Pts',(10.4462775724575,-0.937424827374877,
1.02508498313546));
#18077=CARTESIAN_POINT('Ctrl Pts',(10.4209202812412,-1.01298254961426,1.02648109501254));
#18078=CARTESIAN_POINT('Ctrl Pts',(10.3483173980216,-1.05205297430477,1.02554444431988));
#18079=CARTESIAN_POINT('Ctrl Pts',(10.3053025283406,-1.05463614976313,1.02441711227736));
#18080=CARTESIAN_POINT('',(10.3006295894369,-0.974894988741159,1.1));
#18081=CARTESIAN_POINT('',(10.3053025283406,-1.05463614976313,1.02441711227736));
#18082=CARTESIAN_POINT('Origin',(10.3006295894369,-0.974894988741159,1.02));
#18083=CARTESIAN_POINT('Ctrl Pts',(10.3053025283406,-1.05463614976313,1.02441711227736));
#18084=CARTESIAN_POINT('Ctrl Pts',(10.3483173980216,-1.05205297430477,1.02554444431988));
#18085=CARTESIAN_POINT('Ctrl Pts',(10.4209202812412,-1.01298254961426,1.02648109501254));
#18086=CARTESIAN_POINT('Ctrl Pts',(10.4462775724575,-0.937424827374877,
1.02508498313546));
#18087=CARTESIAN_POINT('Ctrl Pts',(10.4463246402318,-0.905110932257974,
1.02418687649944));
#18088=CARTESIAN_POINT('Ctrl Pts',(10.3664342774515,-0.905110932257974,
1.1));
#18089=CARTESIAN_POINT('Ctrl Pts',(10.3664342774515,-0.920212678972614,
1.1));
#18090=CARTESIAN_POINT('Ctrl Pts',(10.3546350195413,-0.955507038097987,
1.1));
#18091=CARTESIAN_POINT('Ctrl Pts',(10.3207307664069,-0.973717032831462,
1.1));
#18092=CARTESIAN_POINT('Ctrl Pts',(10.3006295894369,-0.974894988741159,
1.1));
#18093=CARTESIAN_POINT('Ctrl Pts',(10.3006295894369,-0.974894988741159,
1.1));
#18094=CARTESIAN_POINT('Ctrl Pts',(8.90133038997308,-1.05689579714676,1.1));
#18095=CARTESIAN_POINT('Ctrl Pts',(5.63386529032775,-1.20659234980357,1.1));
#18096=CARTESIAN_POINT('Ctrl Pts',(2.35953432096223,-1.1387902266302,1.1));
#18097=CARTESIAN_POINT('Ctrl Pts',(0.497468741075922,-0.978719373910683,
1.1));
#18098=CARTESIAN_POINT('Ctrl Pts',(10.3019806204244,-0.997949597787003,
1.1));
#18099=CARTESIAN_POINT('Ctrl Pts',(8.90248440956766,-1.07998148241326,1.10000071389857));
#18100=CARTESIAN_POINT('Ctrl Pts',(5.63428345559727,-1.22975661509925,1.09999860206726));
#18101=CARTESIAN_POINT('Ctrl Pts',(2.35854977485598,-1.16192218645588,1.10000206853834));
#18102=CARTESIAN_POINT('Ctrl Pts',(0.495492436783665,-1.00170924455528,
1.1));
#18103=CARTESIAN_POINT('Ctrl Pts',(10.3043223112023,-1.03790927738781,1.08136574244164));
#18104=CARTESIAN_POINT('Ctrl Pts',(8.90448672538924,-1.11999254202045,1.08133291965814));
#18105=CARTESIAN_POINT('Ctrl Pts',(5.63501252140964,-1.26990499402305,1.08126385742935));
#18106=CARTESIAN_POINT('Ctrl Pts',(2.35683262246169,-1.20200947624765,1.08130376582018));
#18107=CARTESIAN_POINT('Ctrl Pts',(0.492066872450609,-1.0415580073244,1.08139899772624));
#18108=CARTESIAN_POINT('Ctrl Pts',(10.3052465815697,-1.05368144854439,1.04171131144128));
#18109=CARTESIAN_POINT('Ctrl Pts',(8.90527383415966,-1.13574844311122,1.04162635195479));
#18110=CARTESIAN_POINT('Ctrl Pts',(5.63529344743191,-1.28563363803111,1.04144655753461));
#18111=CARTESIAN_POINT('Ctrl Pts',(2.35616768559357,-1.21776439538312,1.04155103737704));
#18112=CARTESIAN_POINT('Ctrl Pts',(0.490711556403977,-1.05732407164794,
1.04179769276967));
#18113=CARTESIAN_POINT('Ctrl Pts',(10.3053025283406,-1.05463614976313,1.02441711227736));
#18114=CARTESIAN_POINT('Ctrl Pts',(8.90532084970199,-1.13668250951809,1.02431679017323));
#18115=CARTESIAN_POINT('Ctrl Pts',(5.63530902077156,-1.28652517622799,1.02410366945797));
#18116=CARTESIAN_POINT('Ctrl Pts',(2.35612886002319,-1.2186808487933,1.02422798328229));
#18117=CARTESIAN_POINT('Ctrl Pts',(0.490627822843887,-1.05829812393464,
1.02451933428366));
#18118=CARTESIAN_POINT('',(0.497468741075922,-0.978719373910683,1.1));
#18119=CARTESIAN_POINT('',(0.490627822843887,-1.05829812393464,1.02451933428366));
#18120=CARTESIAN_POINT('Origin',(0.497468741075922,-0.978719373910683,1.02));
#18121=CARTESIAN_POINT('Ctrl Pts',(0.490627822843887,-1.05829812393464,
1.02451933428366));
#18122=CARTESIAN_POINT('Ctrl Pts',(2.35612886002319,-1.2186808487933,1.02422798328229));
#18123=CARTESIAN_POINT('Ctrl Pts',(5.63530902077156,-1.28652517622799,1.02410366945797));
#18124=CARTESIAN_POINT('Ctrl Pts',(8.90532084970199,-1.13668250951809,1.02431679017323));
#18125=CARTESIAN_POINT('Ctrl Pts',(10.3053025283406,-1.05463614976313,1.02441711227736));
#18126=CARTESIAN_POINT('Ctrl Pts',(10.3006295894369,-0.974894988741159,
1.1));
#18127=CARTESIAN_POINT('Ctrl Pts',(8.90133038997308,-1.05689579714676,1.1));
#18128=CARTESIAN_POINT('Ctrl Pts',(5.63386529032775,-1.20659234980357,1.1));
#18129=CARTESIAN_POINT('Ctrl Pts',(2.35953432096223,-1.1387902266302,1.1));
#18130=CARTESIAN_POINT('Ctrl Pts',(0.497468741075922,-0.978719373910683,
1.1));
#18131=CARTESIAN_POINT('Ctrl Pts',(0.497468741075921,-0.978719373910683,
1.1));
#18132=CARTESIAN_POINT('Ctrl Pts',(0.482693827936028,-0.977449261315989,
1.1));
#18133=CARTESIAN_POINT('Ctrl Pts',(0.449140492346353,-0.963153189418853,
1.1));
#18134=CARTESIAN_POINT('Ctrl Pts',(0.433565722548535,-0.928845297374623,
1.1));
#18135=CARTESIAN_POINT('Ctrl Pts',(0.433565722548535,-0.909072757750428,
1.1));
#18136=CARTESIAN_POINT('Ctrl Pts',(0.495492436783665,-1.00170924455528,
1.1));
#18137=CARTESIAN_POINT('Ctrl Pts',(0.475845599502289,-0.99986336234735,
1.09999428725696));
#18138=CARTESIAN_POINT('Ctrl Pts',(0.431470670910625,-0.980707626108276,
1.09998595101222));
#18139=CARTESIAN_POINT('Ctrl Pts',(0.410656014536328,-0.935396857641307,
1.09999159501496));
#18140=CARTESIAN_POINT('Ctrl Pts',(0.410427643322096,-0.909072757750428,
1.1));
#18141=CARTESIAN_POINT('Ctrl Pts',(0.49206544526959,-1.04157460937658,1.08141381101793));
#18142=CARTESIAN_POINT('Ctrl Pts',(0.464027324938814,-1.03875422423143,
1.08167681576789));
#18143=CARTESIAN_POINT('Ctrl Pts',(0.40089609645214,-1.01114975683443,1.0820463630617));
#18144=CARTESIAN_POINT('Ctrl Pts',(0.370905720538455,-0.946677133941945,
1.08169093175476));
#18145=CARTESIAN_POINT('Ctrl Pts',(0.370309354350992,-0.909072757750428,
1.08130565542949));
#18146=CARTESIAN_POINT('Ctrl Pts',(0.490711556403977,-1.05732407164794,
1.04179769276967));
#18147=CARTESIAN_POINT('Ctrl Pts',(0.459302109313527,-1.05440855600651,
1.04247888820671));
#18148=CARTESIAN_POINT('Ctrl Pts',(0.388222412631637,-1.02376232464153,
1.04344633806995));
#18149=CARTESIAN_POINT('Ctrl Pts',(0.354893537837358,-0.951140796546497,
1.04251250847383));
#18150=CARTESIAN_POINT('Ctrl Pts',(0.354583574894625,-0.909072757750428,
1.0415166534692));
#18151=CARTESIAN_POINT('Ctrl Pts',(0.490627822843887,-1.05829812393464,
1.02451933428366));
#18152=CARTESIAN_POINT('Ctrl Pts',(0.45900946369528,-1.05553438344805,1.02532396689517));
#18153=CARTESIAN_POINT('Ctrl Pts',(0.387169680965019,-1.0248398620393,1.02647307310763));
#18154=CARTESIAN_POINT('Ctrl Pts',(0.353736942373964,-0.951381046565093,
1.02536194261819));
#18155=CARTESIAN_POINT('Ctrl Pts',(0.35367535976817,-0.909072757750428,
1.02418687649944));
#18156=CARTESIAN_POINT('',(0.433565722548535,-0.909072757750428,1.1));
#18157=CARTESIAN_POINT('',(0.35367535976817,-0.909072757750428,1.02418687649944));
#18158=CARTESIAN_POINT('Origin',(0.433565722548536,-0.909072757750428,1.02));
#18159=CARTESIAN_POINT('Ctrl Pts',(0.35367535976817,-0.909072757750428,
1.02418687649944));
#18160=CARTESIAN_POINT('Ctrl Pts',(0.353736942373964,-0.951381046565093,
1.02536194261819));
#18161=CARTESIAN_POINT('Ctrl Pts',(0.387169680965019,-1.0248398620393,1.02647307310763));
#18162=CARTESIAN_POINT('Ctrl Pts',(0.45900946369528,-1.05553438344805,1.02532396689517));
#18163=CARTESIAN_POINT('Ctrl Pts',(0.490627822843887,-1.05829812393464,
1.02451933428366));
#18164=CARTESIAN_POINT('Ctrl Pts',(0.497468741075921,-0.978719373910683,
1.1));
#18165=CARTESIAN_POINT('Ctrl Pts',(0.482693827936028,-0.977449261315989,
1.1));
#18166=CARTESIAN_POINT('Ctrl Pts',(0.449140492346353,-0.963153189418853,
1.1));
#18167=CARTESIAN_POINT('Ctrl Pts',(0.433565722548535,-0.928845297374623,
1.1));
#18168=CARTESIAN_POINT('Ctrl Pts',(0.433565722548535,-0.909072757750428,
1.1));
#18169=CARTESIAN_POINT('Origin',(0.433565722548535,-0.526416499322631,1.02));
#18170=CARTESIAN_POINT('',(0.433565722548535,0.909072757750428,1.1));
#18171=CARTESIAN_POINT('',(0.35367535976817,0.909072757750428,1.02418687649944));
#18172=CARTESIAN_POINT('Origin',(0.433565722548535,0.909072757750428,1.02));
#18173=CARTESIAN_POINT('',(0.35367535976817,-0.526416499322631,1.02418687649944));
#18174=CARTESIAN_POINT('',(0.433565722548535,-0.526416499322631,1.1));
#18175=CARTESIAN_POINT('Ctrl Pts',(0.433565722548535,0.909072757750428,
1.1));
#18176=CARTESIAN_POINT('Ctrl Pts',(0.433565722548535,0.923902162481473,
1.1));
#18177=CARTESIAN_POINT('Ctrl Pts',(0.444925688709976,0.95855828847753,1.1));
#18178=CARTESIAN_POINT('Ctrl Pts',(0.477768856872262,0.977025890449618,
1.1));
#18179=CARTESIAN_POINT('Ctrl Pts',(0.497468741075921,0.978719373910683,
1.1));
#18180=CARTESIAN_POINT('Ctrl Pts',(0.410427643322096,0.909072757750428,
1.1));
#18181=CARTESIAN_POINT('Ctrl Pts',(0.410598921732919,0.928815832685761,
1.09999369626122));
#18182=CARTESIAN_POINT('Ctrl Pts',(0.425924740546693,0.974670094016788,
1.09998538828789));
#18183=CARTESIAN_POINT('Ctrl Pts',(0.469296653719045,0.9992480682759,1.09999238300928));
#18184=CARTESIAN_POINT('Ctrl Pts',(0.495492436783665,1.00170924455528,1.1));
#18185=CARTESIAN_POINT('Ctrl Pts',(0.370309354350991,0.909072757750428,
1.08130565542949));
#18186=CARTESIAN_POINT('Ctrl Pts',(0.370756628991978,0.937276039918598,
1.0815946126737));
#18187=CARTESIAN_POINT('Ctrl Pts',(0.392976709797646,1.00253976529927,1.08203966084696));
#18188=CARTESIAN_POINT('Ctrl Pts',(0.454681284796039,1.03781409584644,1.08176448401818));
#18189=CARTESIAN_POINT('Ctrl Pts',(0.49206544526959,1.04157460937658,1.08141381101793));
#18190=CARTESIAN_POINT('Ctrl Pts',(0.354583574894625,0.909072757750428,
1.0415166534692));
#18191=CARTESIAN_POINT('Ctrl Pts',(0.354816047101877,0.940623786874923,
1.04226354472332));
#18192=CARTESIAN_POINT('Ctrl Pts',(0.379310481833935,1.01405872099116,1.04342813304911));
#18193=CARTESIAN_POINT('Ctrl Pts',(0.448832293580284,1.05343671745598,1.04270595335318));
#18194=CARTESIAN_POINT('Ctrl Pts',(0.490711556403977,1.05732407164794,1.04179769276967));
#18195=CARTESIAN_POINT('Ctrl Pts',(0.35367535976817,0.909072757750428,1.02418687649944));
#18196=CARTESIAN_POINT('Ctrl Pts',(0.353721546722556,0.940803974389028,
1.02506817608927));
#18197=CARTESIAN_POINT('Ctrl Pts',(0.378136805744942,1.01499479618886,1.02645106984513));
#18198=CARTESIAN_POINT('Ctrl Pts',(0.448470010609076,1.05461313661598,1.0255921777666));
#18199=CARTESIAN_POINT('Ctrl Pts',(0.490627822843887,1.05829812393464,1.02451933428366));
#18200=CARTESIAN_POINT('',(0.497468741075921,0.978719373910683,1.1));
#18201=CARTESIAN_POINT('',(0.490627822843887,1.05829812393464,1.02451933428366));
#18202=CARTESIAN_POINT('Origin',(0.497468741075921,0.978719373910683,1.02));
#18203=CARTESIAN_POINT('Ctrl Pts',(0.490627822843887,1.05829812393464,1.02451933428366));
#18204=CARTESIAN_POINT('Ctrl Pts',(0.448470010609076,1.05461313661598,1.0255921777666));
#18205=CARTESIAN_POINT('Ctrl Pts',(0.378136805744942,1.01499479618886,1.02645106984513));
#18206=CARTESIAN_POINT('Ctrl Pts',(0.353721546722556,0.940803974389028,
1.02506817608927));
#18207=CARTESIAN_POINT('Ctrl Pts',(0.35367535976817,0.909072757750428,1.02418687649944));
#18208=CARTESIAN_POINT('Ctrl Pts',(0.433565722548535,0.909072757750428,
1.1));
#18209=CARTESIAN_POINT('Ctrl Pts',(0.433565722548535,0.923902162481473,
1.1));
#18210=CARTESIAN_POINT('Ctrl Pts',(0.444925688709976,0.95855828847753,1.1));
#18211=CARTESIAN_POINT('Ctrl Pts',(0.477768856872262,0.977025890449618,
1.1));
#18212=CARTESIAN_POINT('Ctrl Pts',(0.497468741075921,0.978719373910683,
1.1));
#18213=CARTESIAN_POINT('Ctrl Pts',(0.497468741075922,0.978719373910683,
1.1));
#18214=CARTESIAN_POINT('Ctrl Pts',(1.89401780684616,1.09877250320817,1.1));
#18215=CARTESIAN_POINT('Ctrl Pts',(5.1654052076905,1.21987569230965,1.1));
#18216=CARTESIAN_POINT('Ctrl Pts',(8.43489748265729,1.08422939062092,1.1));
#18217=CARTESIAN_POINT('Ctrl Pts',(10.3006295894369,0.974894988741159,1.1));
#18218=CARTESIAN_POINT('Ctrl Pts',(0.495492436783665,1.00170924455528,1.1));
#18219=CARTESIAN_POINT('Ctrl Pts',(1.89278532112995,1.12186894072949,1.10000155140362));
#18220=CARTESIAN_POINT('Ctrl Pts',(5.16566149651331,1.24305592512388,1.09999870932828));
#18221=CARTESIAN_POINT('Ctrl Pts',(8.43598583180997,1.1073254346241,1.10000095186468));
#18222=CARTESIAN_POINT('Ctrl Pts',(10.3019806204244,0.997949597787003,1.1));
#18223=CARTESIAN_POINT('Ctrl Pts',(0.492066872450609,1.0415580073244,1.08139899772624));
#18224=CARTESIAN_POINT('Ctrl Pts',(1.89064106564166,1.16189659875033,1.08132757380279));
#18225=CARTESIAN_POINT('Ctrl Pts',(5.16610832342906,1.28323142649893,1.0812556832418));
#18226=CARTESIAN_POINT('Ctrl Pts',(8.43787502268472,1.14735362089424,1.08132197873404));
#18227=CARTESIAN_POINT('Ctrl Pts',(10.3043223112023,1.03790927738781,1.08136574244164));
#18228=CARTESIAN_POINT('Ctrl Pts',(0.490711556403977,1.05732407164794,1.04179769276967));
#18229=CARTESIAN_POINT('Ctrl Pts',(1.88980353393473,1.17765430418353,1.04161270124098));
#18230=CARTESIAN_POINT('Ctrl Pts',(5.16628155123749,1.29896165650174,1.04142536433641));
#18231=CARTESIAN_POINT('Ctrl Pts',(8.43861641093843,1.16310409863161,1.04159803213562));
#18232=CARTESIAN_POINT('Ctrl Pts',(10.3052465815697,1.05368144854439,1.04171131144128));
#18233=CARTESIAN_POINT('Ctrl Pts',(0.490627822843887,1.05829812393464,1.02451933428366));
#18234=CARTESIAN_POINT('Ctrl Pts',(1.88975348136405,1.17858515731652,1.02430082105127));
#18235=CARTESIAN_POINT('Ctrl Pts',(5.16629169073646,1.29984841142479,1.02407861909595));
#18236=CARTESIAN_POINT('Ctrl Pts',(8.43866044940558,1.1640312867702,1.02428334948326));
#18237=CARTESIAN_POINT('Ctrl Pts',(10.3053025283406,1.05463614976313,1.02441711227736));
#18238=CARTESIAN_POINT('Ctrl Pts',(10.3053025283406,1.05463614976313,1.02441711227736));
#18239=CARTESIAN_POINT('Ctrl Pts',(8.43866044940558,1.1640312867702,1.02428334948326));
#18240=CARTESIAN_POINT('Ctrl Pts',(5.16629169073646,1.29984841142479,1.02407861909595));
#18241=CARTESIAN_POINT('Ctrl Pts',(1.88975348136405,1.17858515731652,1.02430082105127));
#18242=CARTESIAN_POINT('Ctrl Pts',(0.490627822843887,1.05829812393464,1.02451933428366));
#18243=CARTESIAN_POINT('Ctrl Pts',(0.497468741075922,0.978719373910683,
1.1));
#18244=CARTESIAN_POINT('Ctrl Pts',(1.89401780684616,1.09877250320817,1.1));
#18245=CARTESIAN_POINT('Ctrl Pts',(5.1654052076905,1.21987569230965,1.1));
#18246=CARTESIAN_POINT('Ctrl Pts',(8.43489748265729,1.08422939062092,1.1));
#18247=CARTESIAN_POINT('Ctrl Pts',(10.3006295894369,0.974894988741159,1.1));
#18248=CARTESIAN_POINT('Origin',(0.347167001354737,-1.05283299864526,0.9));
#18249=CARTESIAN_POINT('',(0.347167001354737,0.915565952400859,0.9));
#18250=CARTESIAN_POINT('Ctrl Pts',(0.347167001354737,0.915565952400859,
0.9));
#18251=CARTESIAN_POINT('Ctrl Pts',(0.349336454142569,0.913401548092598,
0.941395625182189));
#18252=CARTESIAN_POINT('Ctrl Pts',(0.351505906947026,0.911237149868421,
0.982791250681617));
#18253=CARTESIAN_POINT('Ctrl Pts',(0.35367535976817,0.909072757750428,1.02418687649944));
#18254=CARTESIAN_POINT('',(0.347167001354737,-0.915565952400859,0.9));
#18255=CARTESIAN_POINT('',(0.347167001354737,-1.05283299864526,0.9));
#18256=CARTESIAN_POINT('Ctrl Pts',(0.35367535976817,-0.909072757750428,
1.02418687649944));
#18257=CARTESIAN_POINT('Ctrl Pts',(0.351505906947026,-0.911237149868421,
0.982791250681617));
#18258=CARTESIAN_POINT('Ctrl Pts',(0.349336454142569,-0.913401548092598,
0.941395625182188));
#18259=CARTESIAN_POINT('Ctrl Pts',(0.347167001354737,-0.915565952400859,
0.9));
#18260=CARTESIAN_POINT('Ctrl Pts',(0.346993933238254,0.915738617787778,
0.896697663613103));
#18261=CARTESIAN_POINT('Ctrl Pts',(0.349221075397351,0.913516658022686,
0.939194067573829));
#18262=CARTESIAN_POINT('Ctrl Pts',(0.351448217573968,0.911294704668933,
0.981690471868858));
#18263=CARTESIAN_POINT('Ctrl Pts',(0.35367535976817,0.909072757750428,1.02418687649944));
#18264=CARTESIAN_POINT('Ctrl Pts',(0.3471095194732,0.958036394339727,0.898903180361322));
#18265=CARTESIAN_POINT('Ctrl Pts',(0.349336694827029,0.955813381999015,
0.941399523267081));
#18266=CARTESIAN_POINT('Ctrl Pts',(0.351563761373338,0.953590428181058,
0.983895874971514));
#18267=CARTESIAN_POINT('Ctrl Pts',(0.353790936839104,0.951367426011707,
1.0263922183879));
#18268=CARTESIAN_POINT('Ctrl Pts',(0.38058410360499,1.03143776743275,0.900986703480571));
#18269=CARTESIAN_POINT('Ctrl Pts',(0.382809509257377,1.02921304595835,0.943483042387942));
#18270=CARTESIAN_POINT('Ctrl Pts',(0.38503494445329,1.0269883029847,0.985979378580875));
#18271=CARTESIAN_POINT('Ctrl Pts',(0.38726034587086,1.02476358729949,1.02847571797107));
#18272=CARTESIAN_POINT('Ctrl Pts',(0.452370958194108,1.06215086202928,0.898830373501354));
#18273=CARTESIAN_POINT('Ctrl Pts',(0.454593549384999,1.0599273359084,0.941326919294252));
#18274=CARTESIAN_POINT('Ctrl Pts',(0.456816159498039,1.05770384366995,0.983823465869045));
#18275=CARTESIAN_POINT('Ctrl Pts',(0.459038739297573,1.0554803259981,1.02632001264655));
#18276=CARTESIAN_POINT('Ctrl Pts',(0.48397786901498,1.06495020962439,0.897320291708494));
#18277=CARTESIAN_POINT('Ctrl Pts',(0.486199596570706,1.06272777115298,0.939816939358577));
#18278=CARTESIAN_POINT('Ctrl Pts',(0.488421317286976,1.06050533819043,0.982313587627294));
#18279=CARTESIAN_POINT('Ctrl Pts',(0.49064303113777,1.05828291075608,1.02481023651688));
#18280=CARTESIAN_POINT('',(0.484117964332956,1.06481006947648,0.9));
#18281=CARTESIAN_POINT('Ctrl Pts',(0.490627822843887,1.05829812393464,1.02451933428366));
#18282=CARTESIAN_POINT('Ctrl Pts',(0.488457876548035,1.06046876718106,0.983012888930867));
#18283=CARTESIAN_POINT('Ctrl Pts',(0.486287923702977,1.06263941570101,0.941506444170341));
#18284=CARTESIAN_POINT('Ctrl Pts',(0.484117964332956,1.06481006947648,0.9));
#18285=CARTESIAN_POINT('Ctrl Pts',(0.484117964332956,1.06481006947648,0.9));
#18286=CARTESIAN_POINT('Ctrl Pts',(0.473400395954556,1.06388989254567,0.899999999998067));
#18287=CARTESIAN_POINT('Ctrl Pts',(0.462835544435656,1.06178983909504,0.899998456484708));
#18288=CARTESIAN_POINT('Ctrl Pts',(0.452598733053303,1.05860868771556,0.899998088469989));
#18289=CARTESIAN_POINT('Ctrl Pts',(0.444242646677269,1.05601198306707,0.899997788067582));
#18290=CARTESIAN_POINT('Ctrl Pts',(0.436104524303727,1.05269365102958,0.899998236040192));
#18291=CARTESIAN_POINT('Ctrl Pts',(0.428287607266336,1.04868302953039,0.899999222960128));
#18292=CARTESIAN_POINT('Ctrl Pts',(0.418720381516706,1.0437743780639,0.900000430864189));
#18293=CARTESIAN_POINT('Ctrl Pts',(0.409734998843702,1.03788190267505,0.900002558923036));
#18294=CARTESIAN_POINT('Ctrl Pts',(0.401509364000825,1.03108161209803,0.900001877425249));
#18295=CARTESIAN_POINT('Ctrl Pts',(0.400282968007853,1.0300677269361,0.900001775817754));
#18296=CARTESIAN_POINT('Ctrl Pts',(0.399073506836177,1.02903357975146,0.900001605039306));
#18297=CARTESIAN_POINT('Ctrl Pts',(0.397881626738084,1.02797933950107,0.900001345423406));
#18298=CARTESIAN_POINT('Ctrl Pts',(0.39256805719391,1.02327938780652,0.900000188019117));
#18299=CARTESIAN_POINT('Ctrl Pts',(0.387603264903844,1.01818054769329,0.899997323013939));
#18300=CARTESIAN_POINT('Ctrl Pts',(0.383010638913681,1.01272978836618,0.899994456107983));
#18301=CARTESIAN_POINT('Ctrl Pts',(0.37606924632558,1.00449139480359,0.899990123005355));
#18302=CARTESIAN_POINT('Ctrl Pts',(0.370046554889952,0.995534526609835,
0.899986018340436));
#18303=CARTESIAN_POINT('Ctrl Pts',(0.3650033874046,0.986038739193365,0.899984773108821));
#18304=CARTESIAN_POINT('Ctrl Pts',(0.361794276996282,0.979996300523246,
0.899983980732651));
#18305=CARTESIAN_POINT('Ctrl Pts',(0.358982518390177,0.973734765189587,
0.899984261914926));
#18306=CARTESIAN_POINT('Ctrl Pts',(0.356593362150852,0.967295151176304,
0.899985518247832));
#18307=CARTESIAN_POINT('Ctrl Pts',(0.352862932284158,0.957240334312622,
0.899987479886722));
#18308=CARTESIAN_POINT('Ctrl Pts',(0.350196128254646,0.946848238515865,
0.899991935314924));
#18309=CARTESIAN_POINT('Ctrl Pts',(0.348668140386249,0.936282377262574,
0.899995621109591));
#18310=CARTESIAN_POINT('Ctrl Pts',(0.347678076093379,0.929436195976283,
0.89999800933123));
#18311=CARTESIAN_POINT('Ctrl Pts',(0.347167001781036,0.922516504287414,
0.899999999966543));
#18312=CARTESIAN_POINT('Ctrl Pts',(0.347167001354737,0.915565952400859,
0.9));
#18313=CARTESIAN_POINT('Ctrl Pts',(0.484117964332956,1.06481006947648,0.9));
#18314=CARTESIAN_POINT('Ctrl Pts',(0.486234267105876,1.06263480888061,0.94150644476122));
#18315=CARTESIAN_POINT('Ctrl Pts',(0.488350569878795,1.06045954828474,0.98301288952244));
#18316=CARTESIAN_POINT('Ctrl Pts',(0.490466872651714,1.05828428768887,1.02451933428366));
#18317=CARTESIAN_POINT('Ctrl Pts',(3.76001591476243,1.34606837492147,0.9));
#18318=CARTESIAN_POINT('Ctrl Pts',(3.76072193310094,1.3438931143256,0.94150644476122));
#18319=CARTESIAN_POINT('Ctrl Pts',(3.76142795143945,1.34171785372973,0.98301288952244));
#18320=CARTESIAN_POINT('Ctrl Pts',(3.76213396977796,1.33954259313386,1.02451933428366));
#18321=CARTESIAN_POINT('Ctrl Pts',(7.03591386519191,1.25287427294368,0.9));
#18322=CARTESIAN_POINT('Ctrl Pts',(7.03520959909601,1.25069901234781,0.94150644476122));
#18323=CARTESIAN_POINT('Ctrl Pts',(7.03450533300011,1.24852375175194,0.98301288952244));
#18324=CARTESIAN_POINT('Ctrl Pts',(7.03380106690421,1.24634849115607,1.02451933428366));
#18325=CARTESIAN_POINT('Ctrl Pts',(10.3118118156214,1.06114656258054,0.9));
#18326=CARTESIAN_POINT('Ctrl Pts',(10.3096972650911,1.05897130198467,0.94150644476122));
#18327=CARTESIAN_POINT('Ctrl Pts',(10.3075827145608,1.0567960413888,0.98301288952244));
#18328=CARTESIAN_POINT('Ctrl Pts',(10.3054681640305,1.05462078079293,1.02451933428366));
#18329=CARTESIAN_POINT('',(10.3118118156214,1.06114656258054,0.9));
#18330=CARTESIAN_POINT('Ctrl Pts',(10.3118118156214,1.06114656258054,0.9));
#18331=CARTESIAN_POINT('Ctrl Pts',(10.3096420485163,1.05897642099582,0.941472370325488));
#18332=CARTESIAN_POINT('Ctrl Pts',(10.3074722860834,1.05680628338526,0.982944741084089));
#18333=CARTESIAN_POINT('Ctrl Pts',(10.3053025283406,1.05463614976313,1.02441711227738));
#18334=CARTESIAN_POINT('Ctrl Pts',(0.484117964332956,1.06481006947648,0.9));
#18335=CARTESIAN_POINT('Ctrl Pts',(3.76001591476244,1.34606837492147,0.9));
#18336=CARTESIAN_POINT('Ctrl Pts',(7.03591386519191,1.25287427294368,0.9));
#18337=CARTESIAN_POINT('Ctrl Pts',(10.3118118156214,1.06114656258054,0.9));
#18338=CARTESIAN_POINT('Ctrl Pts',(10.3119584735067,1.0612932457764,0.897196819041737));
#18339=CARTESIAN_POINT('Ctrl Pts',(10.3097363069231,1.05907069570186,0.939670735378922));
#18340=CARTESIAN_POINT('Ctrl Pts',(10.3075141452397,1.0568481497954,0.982144652170355));
#18341=CARTESIAN_POINT('Ctrl Pts',(10.3052919884757,1.05462560807237,1.02461856941773));
#18342=CARTESIAN_POINT('Ctrl Pts',(10.3549577591382,1.05865952187103,0.899312513938921));
#18343=CARTESIAN_POINT('Ctrl Pts',(10.3527348026837,1.05643589667682,0.941786332790264));
#18344=CARTESIAN_POINT('Ctrl Pts',(10.3505118643323,1.05421236578444,0.984260157591605));
#18345=CARTESIAN_POINT('Ctrl Pts',(10.348288915563,1.05198874626302,1.02673397710222));
#18346=CARTESIAN_POINT('Ctrl Pts',(10.427476572305,1.0195555601276,0.90106705940868));
#18347=CARTESIAN_POINT('Ctrl Pts',(10.4252515051274,1.01733143721131,0.943540744474557));
#18348=CARTESIAN_POINT('Ctrl Pts',(10.423026434404,1.01510729429004,0.986014428272043));
#18349=CARTESIAN_POINT('Ctrl Pts',(10.4208013694594,1.01288317591826,1.02848811366363));
#18350=CARTESIAN_POINT('Ctrl Pts',(10.452914163627,0.944082648463888,0.89845127988914));
#18351=CARTESIAN_POINT('Ctrl Pts',(10.4506882024692,0.941859792143813,0.940924989850352));
#18352=CARTESIAN_POINT('Ctrl Pts',(10.4484622663099,0.939636927142988,0.983398700650476));
#18353=CARTESIAN_POINT('Ctrl Pts',(10.4462363051112,0.937414078664829,1.02587241101113));
#18354=CARTESIAN_POINT('Ctrl Pts',(10.453002503567,0.911777874403687,0.896765653419433));
#18355=CARTESIAN_POINT('Ctrl Pts',(10.4507765491346,0.909555555737009,0.939239394205133));
#18356=CARTESIAN_POINT('Ctrl Pts',(10.4485505946895,0.90733324168256,0.981713135231494));
#18357=CARTESIAN_POINT('Ctrl Pts',(10.4463246402318,0.905110932257975,1.02418687649944));
#18358=CARTESIAN_POINT('',(10.4528329986453,0.911608646352005,0.9));
#18359=CARTESIAN_POINT('Ctrl Pts',(10.4463246402318,0.905110932257975,1.02418687649944));
#18360=CARTESIAN_POINT('Ctrl Pts',(10.4484940930483,0.90727683256362,0.982791250770435));
#18361=CARTESIAN_POINT('Ctrl Pts',(10.4506635458528,0.909442737267073,0.941395625270907));
#18362=CARTESIAN_POINT('Ctrl Pts',(10.4528329986453,0.911608646352005,0.9));
#18363=CARTESIAN_POINT('Ctrl Pts',(10.4528329986453,0.911608646352005,0.9));
#18364=CARTESIAN_POINT('Ctrl Pts',(10.4528329984504,0.922365992175136,0.899999999995018));
#18365=CARTESIAN_POINT('Ctrl Pts',(10.4516419184466,0.933071221555305,0.899998396191737));
#18366=CARTESIAN_POINT('Ctrl Pts',(10.4493455883239,0.943542152407774,0.899997878793429));
#18367=CARTESIAN_POINT('Ctrl Pts',(10.4474685729764,0.952101068966945,0.899997455873155));
#18368=CARTESIAN_POINT('Ctrl Pts',(10.4448518647823,0.96050416098414,0.899997731911133));
#18369=CARTESIAN_POINT('Ctrl Pts',(10.4415172538375,0.968646108261598,0.899998556768105));
#18370=CARTESIAN_POINT('Ctrl Pts',(10.4374420364703,0.978596355981088,0.899999564823172));
#18371=CARTESIAN_POINT('Ctrl Pts',(10.4323389624922,0.988051909949456,0.900001510869465));
#18372=CARTESIAN_POINT('Ctrl Pts',(10.4262707314398,0.996829854811629,0.900000879982417));
#18373=CARTESIAN_POINT('Ctrl Pts',(10.4250393574459,0.998611087749148,0.900000751961929));
#18374=CARTESIAN_POINT('Ctrl Pts',(10.4237680854757,1.0003643483506,0.900000505994341));
#18375=CARTESIAN_POINT('Ctrl Pts',(10.4224572101159,1.00208797543426,0.90000009374416));
#18376=CARTESIAN_POINT('Ctrl Pts',(10.4185057422955,1.00728363107359,0.899998851068177));
#18377=CARTESIAN_POINT('Ctrl Pts',(10.4141947510749,1.0122104380758,0.899996136506224));
#18378=CARTESIAN_POINT('Ctrl Pts',(10.4095592300387,1.01684760353016,0.899993329936423));
#18379=CARTESIAN_POINT('Ctrl Pts',(10.4019420261375,1.02446750958049,0.899988718110854));
#18380=CARTESIAN_POINT('Ctrl Pts',(10.3935294957569,1.03122853977634,0.899984126639313));
#18381=CARTESIAN_POINT('Ctrl Pts',(10.3844977038391,1.03705893037027,0.899982514537369));
#18382=CARTESIAN_POINT('Ctrl Pts',(10.3781912117148,1.04113002863034,0.899981388879436));
#18383=CARTESIAN_POINT('Ctrl Pts',(10.3715817027072,1.04474676663118,0.899981626398985));
#18384=CARTESIAN_POINT('Ctrl Pts',(10.364720849853,1.04787222446317,0.899983147799038));
#18385=CARTESIAN_POINT('Ctrl Pts',(10.3549611185069,1.05231826483487,0.899985312027903));
#18386=CARTESIAN_POINT('Ctrl Pts',(10.34479058664,1.05572789097839,0.899990169054599));
#18387=CARTESIAN_POINT('Ctrl Pts',(10.3343672593286,1.0580160164031,0.899994394012168));
#18388=CARTESIAN_POINT('Ctrl Pts',(10.3269595157814,1.05964216185967,0.899997396642827));
#18389=CARTESIAN_POINT('Ctrl Pts',(10.3194233385871,1.06070108442786,0.899999999979614));
#18390=CARTESIAN_POINT('Ctrl Pts',(10.3118118156214,1.06114656258054,0.9));
#18391=CARTESIAN_POINT('Origin',(5.4,6.06940689584926E-17,1.1));
#18392=CARTESIAN_POINT('Origin',(10.4528329986453,1.05283299864526,0.9));
#18393=CARTESIAN_POINT('',(10.4528329986453,-0.911608646352005,0.9));
#18394=CARTESIAN_POINT('Ctrl Pts',(10.4528329986453,-0.911608646352005,
0.9));
#18395=CARTESIAN_POINT('Ctrl Pts',(10.4506635458528,-0.909442737267072,
0.941395625270908));
#18396=CARTESIAN_POINT('Ctrl Pts',(10.4484940930483,-0.90727683256362,0.982791250770435));
#18397=CARTESIAN_POINT('Ctrl Pts',(10.4463246402318,-0.905110932257974,
1.02418687649944));
#18398=CARTESIAN_POINT('',(10.4528329986453,1.05283299864526,0.9));
#18399=CARTESIAN_POINT('Ctrl Pts',(0.483981659460312,-1.06494641796617,
0.897392794396587));
#18400=CARTESIAN_POINT('Ctrl Pts',(0.486202123526484,-1.0627252433871,0.939865274484676));
#18401=CARTESIAN_POINT('Ctrl Pts',(0.488422580760962,-1.06050407431064,
0.982337755190696));
#18402=CARTESIAN_POINT('Ctrl Pts',(0.49064303113777,-1.05828291075608,1.02481023651688));
#18403=CARTESIAN_POINT('Ctrl Pts',(0.441839113682364,-1.06121395205434,
0.899406236555586));
#18404=CARTESIAN_POINT('Ctrl Pts',(0.444060746976072,-1.05899130022525,
0.941878578466899));
#18405=CARTESIAN_POINT('Ctrl Pts',(0.446282352620465,-1.05676877539366,
0.984350928552248));
#18406=CARTESIAN_POINT('Ctrl Pts',(0.448503975350841,-1.05454613107877,
1.02682327135645));
#18407=CARTESIAN_POINT('Ctrl Pts',(0.371552730979752,-1.02159229167772,
0.901018138383736));
#18408=CARTESIAN_POINT('Ctrl Pts',(0.373777362914204,-1.01936901231721,
0.943490294374253));
#18409=CARTESIAN_POINT('Ctrl Pts',(0.376002007910301,-1.01714569791452,
0.985962447794501));
#18410=CARTESIAN_POINT('Ctrl Pts',(0.378226636819208,-1.01492242480963,
1.02843460423251));
#18411=CARTESIAN_POINT('Ctrl Pts',(0.347084422593646,-0.947458158036175,
0.898424303372123));
#18412=CARTESIAN_POINT('Ctrl Pts',(0.349310306978605,-0.945236691937326,
0.940896495998715));
#18413=CARTESIAN_POINT('Ctrl Pts',(0.351536158132471,-0.943015214174121,
0.983368689735046));
#18414=CARTESIAN_POINT('Ctrl Pts',(0.353762042571371,-0.940793758946387,
1.02584088291578));
#18415=CARTESIAN_POINT('Ctrl Pts',(0.346997732921341,-0.915734826946278,
0.896770165885443));
#18416=CARTESIAN_POINT('Ctrl Pts',(0.349223608519428,-0.913514130802309,
0.939242402422435));
#18417=CARTESIAN_POINT('Ctrl Pts',(0.351449484135017,-0.911293441062403,
0.981714639293352));
#18418=CARTESIAN_POINT('Ctrl Pts',(0.35367535976817,-0.909072757750428,
1.02418687649944));
#18419=CARTESIAN_POINT('',(0.484117964332957,-1.06481006947648,0.9));
#18420=CARTESIAN_POINT('Ctrl Pts',(0.347167001354737,-0.915565952400859,
0.9));
#18421=CARTESIAN_POINT('Ctrl Pts',(0.347167001618251,-0.926324952789844,
0.899999999993398));
#18422=CARTESIAN_POINT('Ctrl Pts',(0.348355267190738,-0.937032860435638,
0.899998616841383));
#18423=CARTESIAN_POINT('Ctrl Pts',(0.350648507770679,-0.947506517879914,
0.899998360166273));
#18424=CARTESIAN_POINT('Ctrl Pts',(0.352522341068277,-0.956064664041459,
0.899998150434084));
#18425=CARTESIAN_POINT('Ctrl Pts',(0.355135157141203,-0.964467130383873,
0.899998666502847));
#18426=CARTESIAN_POINT('Ctrl Pts',(0.358466575399326,-0.972608174091076,
0.89999965996049));
#18427=CARTESIAN_POINT('Ctrl Pts',(0.362538734686669,-0.982559379305286,
0.900000874313493));
#18428=CARTESIAN_POINT('Ctrl Pts',(0.367640276064737,-0.992015301694373,
0.90000291775694));
#18429=CARTESIAN_POINT('Ctrl Pts',(0.373711018494534,-1.00079214745216,
0.900002098461893));
#18430=CARTESIAN_POINT('Ctrl Pts',(0.3746124109217,-1.00209534593109,0.900001976811805));
#18431=CARTESIAN_POINT('Ctrl Pts',(0.375535256028145,-1.00338353399439,
0.900001785555943));
#18432=CARTESIAN_POINT('Ctrl Pts',(0.376479443106529,-1.00465606108108,
0.900001505529245));
#18433=CARTESIAN_POINT('Ctrl Pts',(0.380715143239362,-1.01036472123276,
0.900000249306668));
#18434=CARTESIAN_POINT('Ctrl Pts',(0.38537983051291,-1.01575881671377,0.899997265714102));
#18435=CARTESIAN_POINT('Ctrl Pts',(0.390428509023093,-1.02081078987204,
0.899994288896867));
#18436=CARTESIAN_POINT('Ctrl Pts',(0.398043974952909,-1.02843122547465,
0.899989798642598));
#18437=CARTESIAN_POINT('Ctrl Pts',(0.406453848296673,-1.0351976329321,0.899985566096));
#18438=CARTESIAN_POINT('Ctrl Pts',(0.415484607049401,-1.04103374418621,
0.899984276342262));
#18439=CARTESIAN_POINT('Ctrl Pts',(0.421222938370041,-1.04474213026064,
0.899983456806));
#18440=CARTESIAN_POINT('Ctrl Pts',(0.427212893823217,-1.04807424787086,
0.899983742291921));
#18441=CARTESIAN_POINT('Ctrl Pts',(0.433415948881005,-1.05100146303553,
0.899985033489932));
#18442=CARTESIAN_POINT('Ctrl Pts',(0.443112479013355,-1.05557724541753,
0.899987051872858));
#18443=CARTESIAN_POINT('Ctrl Pts',(0.453235937005982,-1.05912207412747,
0.899991654125809));
#18444=CARTESIAN_POINT('Ctrl Pts',(0.463629957379397,-1.06154692150368,
0.899995467994069));
#18445=CARTESIAN_POINT('Ctrl Pts',(0.470358492676306,-1.06311663856929,
0.899997936889288));
#18446=CARTESIAN_POINT('Ctrl Pts',(0.477201035001208,-1.06421620326297,
0.899999999975707));
#18447=CARTESIAN_POINT('Ctrl Pts',(0.484117964332956,-1.06481006947648,
0.9));
#18448=CARTESIAN_POINT('Ctrl Pts',(0.484117964332957,-1.06481006947648,
0.9));
#18449=CARTESIAN_POINT('Ctrl Pts',(0.486287923702977,-1.06263941570101,
0.941506444170342));
#18450=CARTESIAN_POINT('Ctrl Pts',(0.488457876548035,-1.06046876718106,
0.983012888930867));
#18451=CARTESIAN_POINT('Ctrl Pts',(0.490627822843887,-1.05829812393464,
1.02451933428366));
#18452=CARTESIAN_POINT('Ctrl Pts',(10.453005262311,-0.911780628641664,0.896713013448579));
#18453=CARTESIAN_POINT('Ctrl Pts',(10.4507783882972,-0.909557391891849,
0.939204300891032));
#18454=CARTESIAN_POINT('Ctrl Pts',(10.4485515142709,-0.907334159758067,
0.981695588574342));
#18455=CARTESIAN_POINT('Ctrl Pts',(10.4463246402318,-0.905110932257974,
1.02418687649944));
#18456=CARTESIAN_POINT('Ctrl Pts',(10.4528874757217,-0.954853661617317,
0.898960515458773));
#18457=CARTESIAN_POINT('Ctrl Pts',(10.4506605772126,-0.952629688741643,
0.941451759962203));
#18458=CARTESIAN_POINT('Ctrl Pts',(10.4484337586651,-0.950405759674027,
0.983943010977281));
#18459=CARTESIAN_POINT('Ctrl Pts',(10.4462068600709,-0.94818179413378,1.02643425584837));
#18460=CARTESIAN_POINT('Ctrl Pts',(10.4180804799687,-1.02952167699519,0.901043151378083));
#18461=CARTESIAN_POINT('Ctrl Pts',(10.4158548456208,-1.02729651565793,0.943534394542847));
#18462=CARTESIAN_POINT('Ctrl Pts',(10.413629193759,-1.02507134540722,0.986025636297673));
#18463=CARTESIAN_POINT('Ctrl Pts',(10.4114035625395,-1.02284618829514,1.02851687981561));
#18464=CARTESIAN_POINT('Ctrl Pts',(10.3442106925096,-1.05932070834318,0.898730950115076));
#18465=CARTESIAN_POINT('Ctrl Pts',(10.3419870251366,-1.05709644901815,0.941222341385074));
#18466=CARTESIAN_POINT('Ctrl Pts',(10.3397633429135,-1.0548722146549,0.983713733185165));
#18467=CARTESIAN_POINT('Ctrl Pts',(10.3375396837912,-1.05264796171536,1.0262051251811));
#18468=CARTESIAN_POINT('Ctrl Pts',(10.3119612275562,-1.06129600030118,0.897144178853313));
#18469=CARTESIAN_POINT('Ctrl Pts',(10.309738142952,-1.05907253204827,0.939635641919598));
#18470=CARTESIAN_POINT('Ctrl Pts',(10.3075150632522,-1.05684906796687,0.982127105440503));
#18471=CARTESIAN_POINT('Ctrl Pts',(10.3052919884757,-1.05462560807237,1.02461856941773));
#18472=CARTESIAN_POINT('',(10.3118118156214,-1.06114656258054,0.9));
#18473=CARTESIAN_POINT('Ctrl Pts',(10.3053025283406,-1.05463614976313,1.02441711227736));
#18474=CARTESIAN_POINT('Ctrl Pts',(10.3074722860834,-1.05680628338526,0.982944741084074));
#18475=CARTESIAN_POINT('Ctrl Pts',(10.3096420485163,-1.05897642099582,0.941472370325482));
#18476=CARTESIAN_POINT('Ctrl Pts',(10.3118118156214,-1.06114656258054,0.900000000000001));
#18477=CARTESIAN_POINT('Ctrl Pts',(10.3118118156214,-1.06114656258054,0.900000000000001));
#18478=CARTESIAN_POINT('Ctrl Pts',(10.322549369014,-1.06051812817027,0.899999999998837));
#18479=CARTESIAN_POINT('Ctrl Pts',(10.3331651969327,-1.05870347076406,0.899998279675625));
#18480=CARTESIAN_POINT('Ctrl Pts',(10.3434824690201,-1.05579899810317,0.899997678781422));
#18481=CARTESIAN_POINT('Ctrl Pts',(10.3519099591122,-1.05342652848477,0.899997187951103));
#18482=CARTESIAN_POINT('Ctrl Pts',(10.3601388923794,-1.05032564389788,0.899997411230107));
#18483=CARTESIAN_POINT('Ctrl Pts',(10.368065652211,-1.04652424300033,0.899998227267474));
#18484=CARTESIAN_POINT('Ctrl Pts',(10.3777613500057,-1.04187452040475,0.89999922541197));
#18485=CARTESIAN_POINT('Ctrl Pts',(10.3869029298231,-1.0362271920453,0.900001226887481));
#18486=CARTESIAN_POINT('Ctrl Pts',(10.3953114913929,-1.02965576012812,0.900000692598515));
#18487=CARTESIAN_POINT('Ctrl Pts',(10.3970212347867,-1.0283195669856,0.900000583959597));
#18488=CARTESIAN_POINT('Ctrl Pts',(10.3987005924826,-1.02694501523934,0.900000358370781));
#18489=CARTESIAN_POINT('Ctrl Pts',(10.4003479139729,-1.02553250004787,0.899999966744969));
#18490=CARTESIAN_POINT('Ctrl Pts',(10.4052955867552,-1.02129005981461,0.899998790510468));
#18491=CARTESIAN_POINT('Ctrl Pts',(10.4099546972526,-1.01670546321193,0.899996154952331));
#18492=CARTESIAN_POINT('Ctrl Pts',(10.4143066574475,-1.01181472964029,0.899993423989004));
#18493=CARTESIAN_POINT('Ctrl Pts',(10.4214686344271,-1.00376609875091,0.899988929670213));
#18494=CARTESIAN_POINT('Ctrl Pts',(10.4277268376922,-0.994973664259554,
0.899984438878373));
#18495=CARTESIAN_POINT('Ctrl Pts',(10.4330201329469,-0.985617486073369,
0.899982870029797));
#18496=CARTESIAN_POINT('Ctrl Pts',(10.4367196060238,-0.979078472540647,
0.89998177356478));
#18497=CARTESIAN_POINT('Ctrl Pts',(10.4399470827666,-0.972263038755175,
0.89998201356482));
#18498=CARTESIAN_POINT('Ctrl Pts',(10.4426687152005,-0.965225084739993,
0.899983510148066));
#18499=CARTESIAN_POINT('Ctrl Pts',(10.4465375225522,-0.955220615401818,
0.899985637544916));
#18500=CARTESIAN_POINT('Ctrl Pts',(10.4493477346146,-0.944866529467853,
0.899990392295554));
#18501=CARTESIAN_POINT('Ctrl Pts',(10.4510237312406,-0.934325606572895,
0.899994522211612));
#18502=CARTESIAN_POINT('Ctrl Pts',(10.452215546318,-0.926829869027476,0.899997459029114));
#18503=CARTESIAN_POINT('Ctrl Pts',(10.452832998309,-0.919238945488459,0.899999999973399));
#18504=CARTESIAN_POINT('Ctrl Pts',(10.4528329986453,-0.911608646352004,
0.9));
#18505=CARTESIAN_POINT('Origin',(5.4,0.,0.9));
#18506=CARTESIAN_POINT('Ctrl Pts',(10.3118118156214,-1.06114656258054,0.9));
#18507=CARTESIAN_POINT('Ctrl Pts',(7.03591386519191,-1.25287427294368,0.9));
#18508=CARTESIAN_POINT('Ctrl Pts',(3.76001591476243,-1.34606837492147,0.9));
#18509=CARTESIAN_POINT('Ctrl Pts',(0.484117964332957,-1.06481006947648,
0.9));
#18510=CARTESIAN_POINT('Ctrl Pts',(10.3118118156214,-1.06114656258054,0.9));
#18511=CARTESIAN_POINT('Ctrl Pts',(10.3096972650911,-1.05897130198467,0.94150644476122));
#18512=CARTESIAN_POINT('Ctrl Pts',(10.3075827145608,-1.0567960413888,0.98301288952244));
#18513=CARTESIAN_POINT('Ctrl Pts',(10.3054681640305,-1.05462078079293,1.02451933428366));
#18514=CARTESIAN_POINT('Ctrl Pts',(7.03591386519191,-1.25287427294368,0.9));
#18515=CARTESIAN_POINT('Ctrl Pts',(7.03520959909601,-1.25069901234781,0.94150644476122));
#18516=CARTESIAN_POINT('Ctrl Pts',(7.03450533300011,-1.24852375175194,0.98301288952244));
#18517=CARTESIAN_POINT('Ctrl Pts',(7.03380106690421,-1.24634849115607,1.02451933428366));
#18518=CARTESIAN_POINT('Ctrl Pts',(3.76001591476244,-1.34606837492147,0.9));
#18519=CARTESIAN_POINT('Ctrl Pts',(3.76072193310095,-1.3438931143256,0.94150644476122));
#18520=CARTESIAN_POINT('Ctrl Pts',(3.76142795143946,-1.34171785372973,0.98301288952244));
#18521=CARTESIAN_POINT('Ctrl Pts',(3.76213396977796,-1.33954259313386,1.02451933428366));
#18522=CARTESIAN_POINT('Ctrl Pts',(0.484117964332957,-1.06481006947648,
0.9));
#18523=CARTESIAN_POINT('Ctrl Pts',(0.486234267105876,-1.06263480888061,
0.94150644476122));
#18524=CARTESIAN_POINT('Ctrl Pts',(0.488350569878795,-1.06045954828474,
0.98301288952244));
#18525=CARTESIAN_POINT('Ctrl Pts',(0.490466872651714,-1.05828428768887,
1.02451933428366));
#18566=UNCERTAINTY_MEASURE_WITH_UNIT(LENGTH_MEASURE(0.001),#18581,
'DISTANCE_ACCURACY_VALUE',
'Maximum model space distance between geometric entities at asserted c
onnectivities');
#18568=UNCERTAINTY_MEASURE_WITH_UNIT(LENGTH_MEASURE(0.001),#18581,
'DISTANCE_ACCURACY_VALUE',
'Maximum model space distance between geometric entities at asserted c
onnectivities');
#18578=(
GEOMETRIC_REPRESENTATION_CONTEXT(3)
GLOBAL_UNCERTAINTY_ASSIGNED_CONTEXT((#18566))
GLOBAL_UNIT_ASSIGNED_CONTEXT((#18581,#18583,#18584))
REPRESENTATION_CONTEXT('','3D')
);
#18580=(
GEOMETRIC_REPRESENTATION_CONTEXT(3)
GLOBAL_UNCERTAINTY_ASSIGNED_CONTEXT((#18568))
GLOBAL_UNIT_ASSIGNED_CONTEXT((#18581,#18583,#18584))
REPRESENTATION_CONTEXT('','3D')
);
#18581=(
LENGTH_UNIT()
NAMED_UNIT(*)
SI_UNIT(.CENTI.,.METRE.)
);
#18583=(
NAMED_UNIT(*)
PLANE_ANGLE_UNIT()
SI_UNIT($,.RADIAN.)
);
#18584=(
NAMED_UNIT(*)
SI_UNIT($,.STERADIAN.)
SOLID_ANGLE_UNIT()
);
#18594=SHAPE_DEFINITION_REPRESENTATION(#18605,#18632);
#18605=PRODUCT_DEFINITION_SHAPE('',$,#18644);
#18632=SHAPE_REPRESENTATION('',(#7056),#18578);
#18634=PRODUCT_DEFINITION_CONTEXT('part definition',#18669,'design');
#18644=PRODUCT_DEFINITION('2026-11-10-05-09-36-736','Soft grip layer',#18655,
#18634);
#18655=PRODUCT_DEFINITION_FORMATION('',$,#18680);
#18669=APPLICATION_CONTEXT(
'Core Data for Automotive Mechanical Design Process');
#18670=PRODUCT_CONTEXT('part definition',#18669,'mechanical');
#18680=PRODUCT('2026-11-10-05-09-36-736','Soft grip layer',$,(#18670));
#18688=PRESENTATION_STYLE_ASSIGNMENT((#18696));
#18696=SURFACE_STYLE_USAGE(.BOTH.,#18704);
#18704=SURFACE_SIDE_STYLE('',(#18712));
#18712=SURFACE_STYLE_FILL_AREA(#18720);
#18720=FILL_AREA_STYLE('Sky blue soft grip',(#18728));
#18728=FILL_AREA_STYLE_COLOUR('Sky blue soft grip',#18736);
#18736=COLOUR_RGB('Sky blue soft grip',0.317647058823529,0.686274509803922,
0.890196078431372);
ENDSEC;
END-ISO-10303-21;
